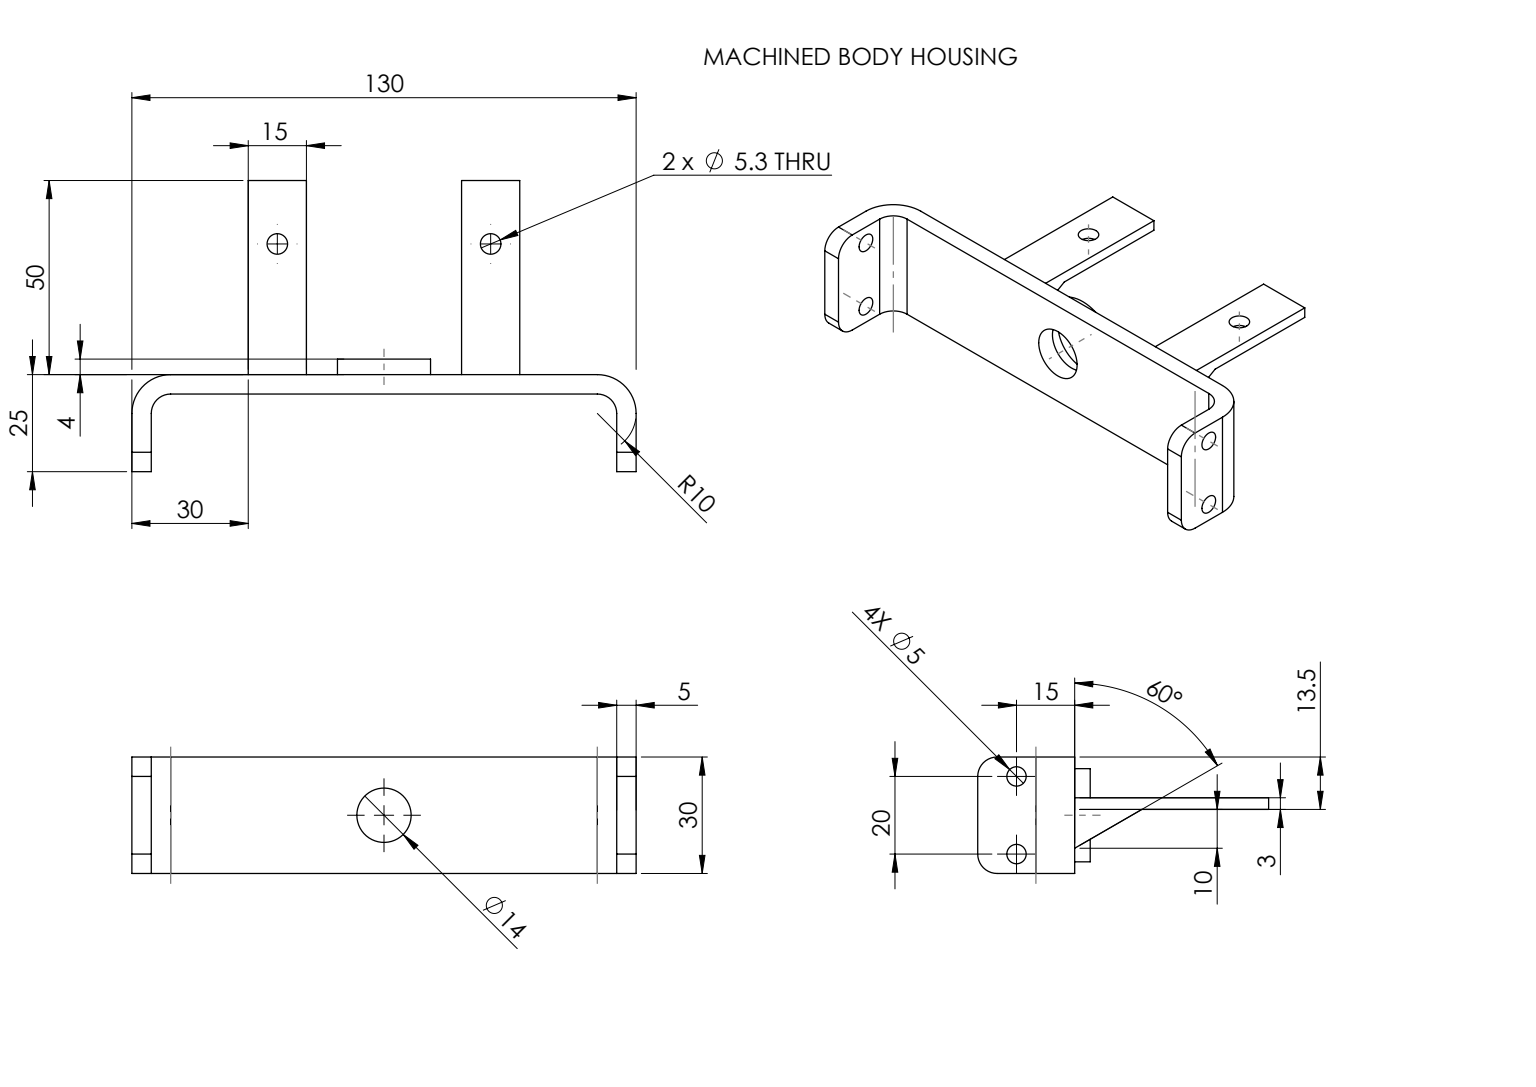
ISO-10303-21;
HEADER;
FILE_DESCRIPTION (('STEP AP214'),
    '1' );
FILE_NAME ('Machined Body Housing.step',
    '2026-10-08T13:46:47',
    ( '' ),
    ( '' ),
    'SwSTEP 2.0',
    'SolidWorks 2026',
    '' );
FILE_SCHEMA (( 'AUTOMOTIVE_DESIGN' ));
ENDSEC;

DATA;
#18=ORIENTED_EDGE ( 'NONE', *, *, #6198, .T. ) ;
#35=DIRECTION ( 'NONE',  ( -1.000000000000000000, 0.000000000000000000, 0.000000000000000000 ) ) ;
#69=PLANE ( 'NONE',  #9969 ) ;
#74=DIRECTION ( 'NONE',  ( 0.000000000000000000, 0.000000000000000000, -1.000000000000000000 ) ) ;
#91=EDGE_CURVE ( 'NONE', #13267, #15347, #17804, .T. ) ;
#103=DIRECTION ( 'NONE',  ( 1.224646799147353207E-16, -0.000000000000000000, 1.000000000000000000 ) ) ;
#106=EDGE_LOOP ( 'NONE', ( #16635, #20382, #2451, #21476 ) ) ;
#112=EDGE_CURVE ( 'NONE', #23518, #15611, #3206, .T. ) ;
#184=ORIENTED_EDGE ( 'NONE', *, *, #1140, .T. ) ;
#197=AXIS2_PLACEMENT_3D ( 'NONE', #16444, #18702, #9272 ) ;
#220=DIRECTION ( 'NONE',  ( 1.000000000000000000, -0.000000000000000000, -0.000000000000000000 ) ) ;
#235=CARTESIAN_POINT ( 'NONE',  ( -4.898587196589412829E-16, 0.000000000000000000, -4.000000000000000000 ) ) ;
#281=ORIENTED_EDGE ( 'NONE', *, *, #12290, .F. ) ;
#288=AXIS2_PLACEMENT_3D ( 'NONE', #14869, #22247, #466 ) ;
#296=DIRECTION ( 'NONE',  ( -0.000000000000000000, -1.000000000000000000, -0.000000000000000000 ) ) ;
#304=ORIENTED_EDGE ( 'NONE', *, *, #3176, .T. ) ;
#329=CARTESIAN_POINT ( 'NONE',  ( 27.50000000000000000, 1.500000000000003109, -33.66025403784446723 ) ) ;
#356=ORIENTED_EDGE ( 'NONE', *, *, #112, .T. ) ;
#362=DIRECTION ( 'NONE',  ( -0.000000000000000000, -1.000000000000000000, -0.000000000000000000 ) ) ;
#374=SHAPE_DEFINITION_REPRESENTATION ( #9332, #13579 ) ;
#392=CARTESIAN_POINT ( 'NONE',  ( -9.000000000000000000, 1.102182119232617714E-15, 1.102182119232617714E-15 ) ) ;
#407=DIRECTION ( 'NONE',  ( 0.000000000000000000, 0.000000000000000000, -1.000000000000000000 ) ) ;
#416=ADVANCED_FACE ( 'NONE', ( #532 ), #16955, .F. ) ;
#430=DIRECTION ( 'NONE',  ( 0.000000000000000000, 0.000000000000000000, -1.000000000000000000 ) ) ;
#463=CARTESIAN_POINT ( 'NONE',  ( 54.99999999999992895, 15.00000000000000000, 1.836970198721037478E-15 ) ) ;
#465=CARTESIAN_POINT ( 'NONE',  ( 9.000000000000000000, 0.000000000000000000, -4.000000000000000888 ) ) ;
#466=DIRECTION ( 'NONE',  ( -1.000000000000000000, 0.000000000000000000, 1.224646799147353207E-16 ) ) ;
#532=FACE_OUTER_BOUND ( 'NONE', #9949, .T. ) ;
#533=DIRECTION ( 'NONE',  ( 0.000000000000000000, 0.000000000000000000, 1.000000000000000000 ) ) ;
#547=EDGE_CURVE ( 'NONE', #15019, #16065, #20991, .T. ) ;
#548=FACE_OUTER_BOUND ( 'NONE', #8173, .T. ) ;
#559=DIRECTION ( 'NONE',  ( 0.000000000000000000, 0.000000000000000000, 1.000000000000000000 ) ) ;
#565=EDGE_LOOP ( 'NONE', ( #20115, #18574, #6373, #5474, #16669 ) ) ;
#589=VERTEX_POINT ( 'NONE', #18015 ) ;
#600=LINE ( 'NONE', #1067, #16099 ) ;
#621=DIRECTION ( 'NONE',  ( -0.000000000000000000, -1.000000000000000000, -0.000000000000000000 ) ) ;
#655=ORIENTED_EDGE ( 'NONE', *, *, #23127, .T. ) ;
#660=VERTEX_POINT ( 'NONE', #8631 ) ;
#677=DIRECTION ( 'NONE',  ( 0.000000000000000000, 0.000000000000000000, -1.000000000000000000 ) ) ;
#690=LINE ( 'NONE', #6575, #22493 ) ;
#693=ORIENTED_EDGE ( 'NONE', *, *, #18920, .T. ) ;
#697=CYLINDRICAL_SURFACE ( 'NONE', #7614, 2.500000000000002220 ) ;
#726=ORIENTED_EDGE ( 'NONE', *, *, #16884, .F. ) ;
#731=EDGE_LOOP ( 'NONE', ( #13217, #18222 ) ) ;
#733=EDGE_LOOP ( 'NONE', ( #2981, #9011 ) ) ;
#744=CYLINDRICAL_SURFACE ( 'NONE', #19501, 4.999999999999996447 ) ;
#754=VECTOR ( 'NONE', #8335, 1000.000000000000000 ) ;
#766=LINE ( 'NONE', #2680, #12959 ) ;
#770=VECTOR ( 'NONE', #3245, 1000.000000000000000 ) ;
#771=DIRECTION ( 'NONE',  ( 1.000000000000000000, 0.000000000000000000, 1.040834085586083271E-15 ) ) ;
#792=ORIENTED_EDGE ( 'NONE', *, *, #18099, .T. ) ;
#809=CARTESIAN_POINT ( 'NONE',  ( -65.00000000000000000, 9.999999999999998224, 14.99999999999999645 ) ) ;
#811=ORIENTED_EDGE ( 'NONE', *, *, #17044, .F. ) ;
#814=PLANE ( 'NONE',  #15172 ) ;
#831=DIRECTION ( 'NONE',  ( -1.000000000000000000, 0.000000000000000000, 1.239088197126290817E-16 ) ) ;
#897=ORIENTED_EDGE ( 'NONE', *, *, #13576, .T. ) ;
#900=DIRECTION ( 'NONE',  ( 1.000000000000000000, -0.000000000000000000, -1.224646799147353454E-16 ) ) ;
#912=CYLINDRICAL_SURFACE ( 'NONE', #1944, 5.000000000000000888 ) ;
#937=DIRECTION ( 'NONE',  ( 1.000000000000000000, 0.000000000000000000, 0.000000000000000000 ) ) ;
#941=VECTOR ( 'NONE', #12912, 1000.000000000000000 ) ;
#942=CARTESIAN_POINT ( 'NONE',  ( 54.99999999999994316, -8.499999999999944933, 1.836970198721036294E-15 ) ) ;
#954=EDGE_LOOP ( 'NONE', ( #23586, #9037, #13919, #18797 ) ) ;
#956=ORIENTED_EDGE ( 'NONE', *, *, #4066, .T. ) ;
#979=ORIENTED_EDGE ( 'NONE', *, *, #3064, .F. ) ;
#1004=EDGE_CURVE ( 'NONE', #5469, #15347, #8225, .T. ) ;
#1037=EDGE_CURVE ( 'NONE', #23404, #17536, #10992, .T. ) ;
#1043=ORIENTED_EDGE ( 'NONE', *, *, #13376, .T. ) ;
#1058=CARTESIAN_POINT ( 'NONE',  ( 65.00000000000000000, 9.999999999999998224, 19.99999999999999645 ) ) ;
#1061=LINE ( 'NONE', #942, #17401 ) ;
#1067=CARTESIAN_POINT ( 'NONE',  ( 54.99999999999992895, 15.00000000000000000, 1.836970198721037478E-15 ) ) ;
#1075=ORIENTED_EDGE ( 'NONE', *, *, #7209, .F. ) ;
#1081=LINE ( 'NONE', #13691, #1932 ) ;
#1094=ORIENTED_EDGE ( 'NONE', *, *, #6571, .T. ) ;
#1099=VECTOR ( 'NONE', #15927, 1000.000000000000000 ) ;
#1104=ORIENTED_EDGE ( 'NONE', *, *, #9994, .F. ) ;
#1133=CARTESIAN_POINT ( 'NONE',  ( -20.00000000000001066, 4.500000000000003553, -50.00000000000000000 ) ) ;
#1140=EDGE_CURVE ( 'NONE', #11837, #5919, #23282, .T. ) ;
#1143=AXIS2_PLACEMENT_3D ( 'NONE', #12271, #5410, #7224 ) ;
#1156=DIRECTION ( 'NONE',  ( 1.000000000000000000, -0.000000000000000000, -0.000000000000000000 ) ) ;
#1159=CARTESIAN_POINT ( 'NONE',  ( 60.00000000000000711, -15.00000000000000000, 19.99999999999999645 ) ) ;
#1201=EDGE_CURVE ( 'NONE', #19518, #3871, #23160, .T. ) ;
#1210=LINE ( 'NONE', #8194, #8825 ) ;
#1237=ORIENTED_EDGE ( 'NONE', *, *, #15576, .F. ) ;
#1268=LINE ( 'NONE', #10304, #1617 ) ;
#1284=CARTESIAN_POINT ( 'NONE',  ( 65.00000000000000000, -9.999999999999998224, 19.99999999999999645 ) ) ;
#1297=VERTEX_POINT ( 'NONE', #7729 ) ;
#1305=ORIENTED_EDGE ( 'NONE', *, *, #8806, .T. ) ;
#1313=DIRECTION ( 'NONE',  ( 1.000000000000000000, 0.000000000000000000, 0.000000000000000000 ) ) ;
#1320=DIRECTION ( 'NONE',  ( 1.224646799147353207E-16, -0.000000000000000000, 1.000000000000000000 ) ) ;
#1357=VERTEX_POINT ( 'NONE', #22052 ) ;
#1379=LINE ( 'NONE', #7284, #5572 ) ;
#1382=PLANE ( 'NONE',  #19705 ) ;
#1426=AXIS2_PLACEMENT_3D ( 'NONE', #20889, #22335, #13514 ) ;
#1431=DIRECTION ( 'NONE',  ( 1.224646799147353207E-16, -0.000000000000000000, 1.000000000000000000 ) ) ;
#1462=EDGE_CURVE ( 'NONE', #20146, #12336, #3240, .T. ) ;
#1464=CARTESIAN_POINT ( 'NONE',  ( 20.00000000000000000, 1.500000000000003109, -17.32050807568893092 ) ) ;
#1471=EDGE_CURVE ( 'NONE', #16384, #8981, #8772, .T. ) ;
#1475=AXIS2_PLACEMENT_3D ( 'NONE', #8775, #10591, #19885 ) ;
#1498=CIRCLE ( 'NONE', #10721, 2.499999999999998668 ) ;
#1514=DIRECTION ( 'NONE',  ( 1.000000000000000000, 4.625929269271486900E-16, 0.000000000000000000 ) ) ;
#1520=ORIENTED_EDGE ( 'NONE', *, *, #23567, .F. ) ;
#1528=DIRECTION ( 'NONE',  ( -1.224646799147353207E-16, 0.000000000000000000, -1.000000000000000000 ) ) ;
#1542=( NAMED_UNIT ( * ) PLANE_ANGLE_UNIT ( ) SI_UNIT ( $, .RADIAN. ) );
#1561=DIRECTION ( 'NONE',  ( -1.000000000000000000, 0.000000000000000000, 0.000000000000000000 ) ) ;
#1569=ADVANCED_FACE ( 'NONE', ( #21794 ), #6968, .T. ) ;
#1582=ADVANCED_FACE ( 'NONE', ( #23477 ), #14407, .F. ) ;
#1585=CARTESIAN_POINT ( 'NONE',  ( -20.00000000000001066, 4.500000000000003553, -50.00000000000000000 ) ) ;
#1617=VECTOR ( 'NONE', #1156, 1000.000000000000000 ) ;
#1626=CARTESIAN_POINT ( 'NONE',  ( -65.00000000000000000, 9.999999999999998224, 25.00000000000001421 ) ) ;
#1630=CARTESIAN_POINT ( 'NONE',  ( 65.00000000000000000, 15.00000000000000000, 10.00000000000007105 ) ) ;
#1633=LINE ( 'NONE', #12448, #22458 ) ;
#1662=FACE_OUTER_BOUND ( 'NONE', #23691, .T. ) ;
#1670=VECTOR ( 'NONE', #16250, 1000.000000000000000 ) ;
#1675=ADVANCED_FACE ( 'NONE', ( #12532 ), #16223, .F. ) ;
#1682=DIRECTION ( 'NONE',  ( -1.000000000000000000, 0.000000000000000000, 1.224646799147353207E-16 ) ) ;
#1694=CYLINDRICAL_SURFACE ( 'NONE', #12537, 2.649999999999999467 ) ;
#1722=CARTESIAN_POINT ( 'NONE',  ( -54.99999999999992895, 15.00000000000000000, 5.000000000000015987 ) ) ;
#1725=PLANE ( 'NONE',  #11097 ) ;
#1726=CARTESIAN_POINT ( 'NONE',  ( 55.00000000000000711, 15.00000000000000000, 10.00000000000000000 ) ) ;
#1730=EDGE_CURVE ( 'NONE', #18272, #11666, #15988, .T. ) ;
#1739=EDGE_CURVE ( 'NONE', #7101, #5362, #20376, .T. ) ;
#1747=DIRECTION ( 'NONE',  ( 0.000000000000000000, 0.000000000000000000, 1.000000000000000000 ) ) ;
#1748=CARTESIAN_POINT ( 'NONE',  ( 65.00000000000000000, -10.00000000000000178, 12.49999999999999467 ) ) ;
#1750=ORIENTED_EDGE ( 'NONE', *, *, #9693, .F. ) ;
#1767=DIRECTION ( 'NONE',  ( 1.224646799147353207E-16, -0.000000000000000000, 1.000000000000000000 ) ) ;
#1789=CARTESIAN_POINT ( 'NONE',  ( -4.898587196589412829E-16, 0.000000000000000000, -4.000000000000000000 ) ) ;
#1796=CARTESIAN_POINT ( 'NONE',  ( -35.00000000000000000, 4.500000000000003553, 4.286263797015736496E-15 ) ) ;
#1813=DIRECTION ( 'NONE',  ( 0.000000000000000000, 0.000000000000000000, -1.000000000000000000 ) ) ;
#1840=ORIENTED_EDGE ( 'NONE', *, *, #8806, .F. ) ;
#1841=FACE_OUTER_BOUND ( 'NONE', #21249, .T. ) ;
#1844=EDGE_CURVE ( 'NONE', #13106, #19458, #9139, .T. ) ;
#1850=CARTESIAN_POINT ( 'NONE',  ( -54.99999999999992895, 15.00000000000000000, 5.000000000000015987 ) ) ;
#1866=VECTOR ( 'NONE', #21905, 1000.000000000000000 ) ;
#1873=EDGE_CURVE ( 'NONE', #19365, #1924, #15036, .T. ) ;
#1879=DIRECTION ( 'NONE',  ( -1.000000000000000000, 0.000000000000000000, 9.637352644315595243E-17 ) ) ;
#1889=AXIS2_PLACEMENT_3D ( 'NONE', #22318, #533, #7508 ) ;
#1913=VERTEX_POINT ( 'NONE', #16458 ) ;
#1919=DIRECTION ( 'NONE',  ( -1.000000000000000000, 0.000000000000000000, 1.445602896647339163E-16 ) ) ;
#1924=VERTEX_POINT ( 'NONE', #392 ) ;
#1929=PRODUCT_CONTEXT ( 'NONE', #12856, 'mechanical' ) ;
#1930=DIRECTION ( 'NONE',  ( -1.224646799147353207E-16, 0.000000000000000000, -1.000000000000000000 ) ) ;
#1932=VECTOR ( 'NONE', #20953, 1000.000000000000000 ) ;
#1933=ORIENTED_EDGE ( 'NONE', *, *, #10842, .F. ) ;
#1944=AXIS2_PLACEMENT_3D ( 'NONE', #8248, #20792, #13523 ) ;
#1961=CARTESIAN_POINT ( 'NONE',  ( -4.898587196589412829E-16, 0.000000000000000000, -4.000000000000000000 ) ) ;
#1962=CARTESIAN_POINT ( 'NONE',  ( 20.00000000000000355, 4.500000000000003553, -2.449293598294706907E-15 ) ) ;
#1967=CARTESIAN_POINT ( 'NONE',  ( -27.50000000000000711, 1.500000000000003109, -31.01025403784446510 ) ) ;
#1979=EDGE_LOOP ( 'NONE', ( #21980, #9928, #1104, #8440 ) ) ;
#1997=DIRECTION ( 'NONE',  ( 0.000000000000000000, 0.000000000000000000, 1.000000000000000000 ) ) ;
#2012=LINE ( 'NONE', #16764, #18322 ) ;
#2017=DIRECTION ( 'NONE',  ( 0.000000000000000000, 0.000000000000000000, -1.000000000000000000 ) ) ;
#2020=VERTEX_POINT ( 'NONE', #8302 ) ;
#2023=CARTESIAN_POINT ( 'NONE',  ( -60.00000000000000711, -15.00000000000000000, 10.00000000000004974 ) ) ;
#2069=DIRECTION ( 'NONE',  ( 0.000000000000000000, 0.000000000000000000, 1.000000000000000000 ) ) ;
#2100=ORIENTED_EDGE ( 'NONE', *, *, #3101, .T. ) ;
#2111=AXIS2_PLACEMENT_3D ( 'NONE', #14632, #9595, #21892 ) ;
#2141=ADVANCED_FACE ( 'NONE', ( #6972 ), #5163, .F. ) ;
#2155=EDGE_LOOP ( 'NONE', ( #7268, #12154, #13017, #8583 ) ) ;
#2203=AXIS2_PLACEMENT_3D ( 'NONE', #4413, #11869, #6458 ) ;
#2223=DIRECTION ( 'NONE',  ( -0.000000000000000000, -1.000000000000000000, -0.000000000000000000 ) ) ;
#2236=VERTEX_POINT ( 'NONE', #7003 ) ;
#2271=DIRECTION ( 'NONE',  ( 0.000000000000000000, 0.000000000000000000, -1.000000000000000000 ) ) ;
#2290=EDGE_LOOP ( 'NONE', ( #6796, #9438 ) ) ;
#2329=LINE ( 'NONE', #7976, #16409 ) ;
#2351=LINE ( 'NONE', #15558, #6078 ) ;
#2372=VERTEX_POINT ( 'NONE', #4318 ) ;
#2389=DIRECTION ( 'NONE',  ( 1.000000000000000000, 0.000000000000000000, 0.000000000000000000 ) ) ;
#2406=EDGE_LOOP ( 'NONE', ( #2495, #956 ) ) ;
#2426=ORIENTED_EDGE ( 'NONE', *, *, #14982, .T. ) ;
#2451=ORIENTED_EDGE ( 'NONE', *, *, #3652, .F. ) ;
#2467=VECTOR ( 'NONE', #12355, 1000.000000000000000 ) ;
#2495=ORIENTED_EDGE ( 'NONE', *, *, #15806, .T. ) ;
#2511=DIRECTION ( 'NONE',  ( 0.000000000000000000, 0.000000000000000000, 1.000000000000000000 ) ) ;
#2536=DIRECTION ( 'NONE',  ( 1.224646799147353207E-16, -0.000000000000000000, 1.000000000000000000 ) ) ;
#2539=ORIENTED_EDGE ( 'NONE', *, *, #16677, .T. ) ;
#2560=PLANE ( 'NONE',  #21397 ) ;
#2586=CARTESIAN_POINT ( 'NONE',  ( -20.00000000000000711, 1.500000000000003109, -17.32050807568893092 ) ) ;
#2609=CIRCLE ( 'NONE', #5678, 2.500000000000000444 ) ;
#2633=DIRECTION ( 'NONE',  ( 0.000000000000000000, -1.000000000000000000, 0.000000000000000000 ) ) ;
#2634=PRODUCT ( 'Machined Body Housing', 'Machined Body Housing', '', ( #1929 ) ) ;
#2650=AXIS2_PLACEMENT_3D ( 'NONE', #8276, #2970, #4899 ) ;
#2673=ORIENTED_EDGE ( 'NONE', *, *, #17745, .F. ) ;
#2680=CARTESIAN_POINT ( 'NONE',  ( 34.99999999999999289, 16.40063509461080571, -43.12916512459904794 ) ) ;
#2701=VERTEX_POINT ( 'NONE', #12627 ) ;
#2704=LINE ( 'NONE', #18874, #16750 ) ;
#2721=CARTESIAN_POINT ( 'NONE',  ( 60.00000000000000000, 9.999999999999998224, 14.99999999999999645 ) ) ;
#2722=DIRECTION ( 'NONE',  ( 0.000000000000000000, 0.000000000000000000, -1.000000000000000000 ) ) ;
#2725=DIRECTION ( 'NONE',  ( -1.224646799147353207E-16, 0.000000000000000000, -1.000000000000000000 ) ) ;
#2736=EDGE_CURVE ( 'NONE', #15611, #13122, #20088, .T. ) ;
#2753=CARTESIAN_POINT ( 'NONE',  ( 20.00000000000000355, 4.500000000000003553, -2.449293598294706907E-15 ) ) ;
#2765=CIRCLE ( 'NONE', #11983, 2.500000000000000444 ) ;
#2802=CARTESIAN_POINT ( 'NONE',  ( -65.00000000000000000, 15.00000000000000000, 10.00000000000008882 ) ) ;
#2832=LINE ( 'NONE', #6210, #21016 ) ;
#2845=CIRCLE ( 'NONE', #14351, 7.000000000000000000 ) ;
#2852=CYLINDRICAL_SURFACE ( 'NONE', #16801, 5.000000000000000888 ) ;
#2863=CARTESIAN_POINT ( 'NONE',  ( -20.00000000000000355, 4.500000000000003553, 2.449293598294706907E-15 ) ) ;
#2872=ORIENTED_EDGE ( 'NONE', *, *, #10537, .F. ) ;
#2883=CIRCLE ( 'NONE', #5960, 2.500000000000000444 ) ;
#2884=VECTOR ( 'NONE', #10996, 1000.000000000000000 ) ;
#2902=EDGE_LOOP ( 'NONE', ( #16031, #23184 ) ) ;
#2912=CARTESIAN_POINT ( 'NONE',  ( -20.00000000000001066, 4.500000000000003553, -50.00000000000000000 ) ) ;
#2939=DIRECTION ( 'NONE',  ( -1.000000000000000000, 0.000000000000000000, 0.000000000000000000 ) ) ;
#2967=VERTEX_POINT ( 'NONE', #10539 ) ;
#2970=DIRECTION ( 'NONE',  ( -1.224646799147353207E-16, 0.000000000000000000, -1.000000000000000000 ) ) ;
#2971=DIRECTION ( 'NONE',  ( 4.625929269271486900E-16, -1.000000000000000000, -5.665129472695380173E-32 ) ) ;
#2974=DIRECTION ( 'NONE',  ( 1.224646799147353207E-16, -0.000000000000000000, 1.000000000000000000 ) ) ;
#2976=ORIENTED_EDGE ( 'NONE', *, *, #19049, .T. ) ;
#2981=ORIENTED_EDGE ( 'NONE', *, *, #3861, .T. ) ;
#2990=VERTEX_POINT ( 'NONE', #17473 ) ;
#2999=CIRCLE ( 'NONE', #8002, 5.000000000000004441 ) ;
#3032=DIRECTION ( 'NONE',  ( -1.000000000000000000, -4.625929269271486900E-16, 1.224646799147353207E-16 ) ) ;
#3034=EDGE_CURVE ( 'NONE', #11666, #22477, #2765, .T. ) ;
#3043=EDGE_CURVE ( 'NONE', #9561, #17175, #8918, .T. ) ;
#3044=CARTESIAN_POINT ( 'NONE',  ( -6.123233995736766085E-15, 0.000000000000000000, -50.00000000000000000 ) ) ;
#3048=DIRECTION ( 'NONE',  ( 1.224646799147353207E-16, -0.000000000000000000, 1.000000000000000000 ) ) ;
#3060=CIRCLE ( 'NONE', #9211, 2.500000000000000444 ) ;
#3062=UNCERTAINTY_MEASURE_WITH_UNIT (LENGTH_MEASURE( 1.000000000000000082E-05 ), #21533, 'distance_accuracy_value', 'NONE');
#3064=EDGE_CURVE ( 'NONE', #21915, #22477, #1268, .T. ) ;
#3085=CARTESIAN_POINT ( 'NONE',  ( 60.00000000000000711, 15.00000000000000000, 10.00000000000007105 ) ) ;
#3088=ORIENTED_EDGE ( 'NONE', *, *, #20465, .T. ) ;
#3101=EDGE_CURVE ( 'NONE', #17422, #16065, #23187, .T. ) ;
#3107=ORIENTED_EDGE ( 'NONE', *, *, #19599, .F. ) ;
#3111=CARTESIAN_POINT ( 'NONE',  ( 0.000000000000000000, 0.000000000000000000, 0.000000000000000000 ) ) ;
#3119=CARTESIAN_POINT ( 'NONE',  ( -4.898587196589412829E-16, 0.000000000000000000, -4.000000000000000000 ) ) ;
#3161=ORIENTED_EDGE ( 'NONE', *, *, #22071, .T. ) ;
#3176=EDGE_CURVE ( 'NONE', #9843, #3750, #11234, .T. ) ;
#3188=CARTESIAN_POINT ( 'NONE',  ( 54.99999999999996447, 15.00000000000000000, 5.000000000000003553 ) ) ;
#3206=CIRCLE ( 'NONE', #20788, 10.00000000000000178 ) ;
#3240=LINE ( 'NONE', #5156, #6403 ) ;
#3245=DIRECTION ( 'NONE',  ( 1.000000000000000000, -0.000000000000000000, -0.000000000000000000 ) ) ;
#3252=EDGE_LOOP ( 'NONE', ( #9859, #14478 ) ) ;
#3260=DIRECTION ( 'NONE',  ( 4.625929269271486900E-16, -1.000000000000000000, -5.665129472695380173E-32 ) ) ;
#3261=VECTOR ( 'NONE', #12153, 1000.000000000000000 ) ;
#3263=AXIS2_PLACEMENT_3D ( 'NONE', #15448, #22715, #20682 ) ;
#3271=AXIS2_PLACEMENT_3D ( 'NONE', #809, #13421, #2722 ) ;
#3284=DIRECTION ( 'NONE',  ( 1.000000000000000000, 4.625929269271485914E-16, -1.224646799147353454E-16 ) ) ;
#3293=DIRECTION ( 'NONE',  ( -1.224646799147353207E-16, 0.000000000000000000, -1.000000000000000000 ) ) ;
#3323=VECTOR ( 'NONE', #3284, 1000.000000000000000 ) ;
#3338=VECTOR ( 'NONE', #14817, 1000.000000000000000 ) ;
#3353=CARTESIAN_POINT ( 'NONE',  ( 0.000000000000000000, 0.000000000000000000, 1.734723475976807094E-15 ) ) ;
#3381=CARTESIAN_POINT ( 'NONE',  ( 19.99999999999999645, 4.500000000000003553, -50.00000000000000000 ) ) ;
#3382=ORIENTED_EDGE ( 'NONE', *, *, #11929, .T. ) ;
#3383=CARTESIAN_POINT ( 'NONE',  ( -65.00000000000000000, 9.999999999999998224, 12.49999999999999289 ) ) ;
#3399=EDGE_CURVE ( 'NONE', #17589, #22866, #10576, .T. ) ;
#3418=FACE_OUTER_BOUND ( 'NONE', #19840, .T. ) ;
#3434=DIRECTION ( 'NONE',  ( 1.000000000000000000, 0.000000000000000000, -1.224646799147353207E-16 ) ) ;
#3452=CARTESIAN_POINT ( 'NONE',  ( 65.00000000000000000, 9.999999999999998224, 14.99999999999999645 ) ) ;
#3464=ORIENTED_EDGE ( 'NONE', *, *, #6828, .F. ) ;
#3489=DIRECTION ( 'NONE',  ( -1.000000000000000000, 0.000000000000000000, 0.000000000000000000 ) ) ;
#3495=APPLICATION_CONTEXT ( 'automotive_design' ) ;
#3507=DIRECTION ( 'NONE',  ( -0.000000000000000000, -0.000000000000000000, 1.000000000000000000 ) ) ;
#3524=EDGE_LOOP ( 'NONE', ( #18220, #11976 ) ) ;
#3530=ORIENTED_EDGE ( 'NONE', *, *, #6636, .T. ) ;
#3557=EDGE_LOOP ( 'NONE', ( #3991, #655 ) ) ;
#3561=ADVANCED_FACE ( 'NONE', ( #7547, #10918 ), #11268, .T. ) ;
#3570=DIRECTION ( 'NONE',  ( 1.000000000000000000, -0.000000000000000000, -0.000000000000000000 ) ) ;
#3609=DIRECTION ( 'NONE',  ( 1.000000000000000000, 0.000000000000000000, -1.224646799147353207E-16 ) ) ;
#3612=DIRECTION ( 'NONE',  ( -0.000000000000000000, -0.000000000000000000, 1.000000000000000000 ) ) ;
#3616=AXIS2_PLACEMENT_3D ( 'NONE', #20348, #19888, #3489 ) ;
#3650=LINE ( 'NONE', #1850, #21769 ) ;
#3652=EDGE_CURVE ( 'NONE', #7101, #9090, #22392, .T. ) ;
#3656=AXIS2_PLACEMENT_3D ( 'NONE', #21284, #10210, #2511 ) ;
#3657=DIRECTION ( 'NONE',  ( 0.000000000000000000, 0.000000000000000000, 1.000000000000000000 ) ) ;
#3659=DIRECTION ( 'NONE',  ( 0.000000000000000000, -0.000000000000000000, 1.000000000000000000 ) ) ;
#3663=ORIENTED_EDGE ( 'NONE', *, *, #1140, .F. ) ;
#3666=CARTESIAN_POINT ( 'NONE',  ( 20.00000000000000000, 1.500000000000003109, -17.32050807568893092 ) ) ;
#3682=CARTESIAN_POINT ( 'NONE',  ( -20.00000000000000711, 1.500000000000003109, -17.32050807568893092 ) ) ;
#3688=EDGE_CURVE ( 'NONE', #11955, #2020, #16528, .T. ) ;
#3728=CARTESIAN_POINT ( 'NONE',  ( 7.000000000000000000, 0.000000000000000000, 1.734723475976807094E-15 ) ) ;
#3743=VERTEX_POINT ( 'NONE', #4650 ) ;
#3750=VERTEX_POINT ( 'NONE', #20914 ) ;
#3769=LINE ( 'NONE', #15301, #16820 ) ;
#3776=CARTESIAN_POINT ( 'NONE',  ( 19.99999999999999645, 1.500000000000003109, -50.00000000000000000 ) ) ;
#3800=ADVANCED_FACE ( 'NONE', ( #22968 ), #814, .T. ) ;
#3808=AXIS2_PLACEMENT_3D ( 'NONE', #3452, #17945, #14727 ) ;
#3831=DIRECTION ( 'NONE',  ( -0.000000000000000000, -1.000000000000000000, -0.000000000000000000 ) ) ;
#3836=VECTOR ( 'NONE', #1682, 1000.000000000000000 ) ;
#3861=EDGE_CURVE ( 'NONE', #22477, #11666, #2883, .T. ) ;
#3871=VERTEX_POINT ( 'NONE', #15580 ) ;
#3894=EDGE_CURVE ( 'NONE', #7429, #13541, #9042, .T. ) ;
#3896=ORIENTED_EDGE ( 'NONE', *, *, #4429, .T. ) ;
#3912=VERTEX_POINT ( 'NONE', #23322 ) ;
#3922=EDGE_LOOP ( 'NONE', ( #18403, #14686, #11774, #18278 ) ) ;
#3927=AXIS2_PLACEMENT_3D ( 'NONE', #13450, #22511, #22024 ) ;
#3944=CARTESIAN_POINT ( 'NONE',  ( 60.00000000000000000, -10.00000000000000178, 14.99999999999999467 ) ) ;
#3962=ORIENTED_EDGE ( 'NONE', *, *, #23567, .T. ) ;
#3991=ORIENTED_EDGE ( 'NONE', *, *, #9236, .T. ) ;
#4001=CIRCLE ( 'NONE', #5146, 2.649999999999999467 ) ;
#4012=VECTOR ( 'NONE', #21254, 1000.000000000000000 ) ;
#4016=CARTESIAN_POINT ( 'NONE',  ( 54.99999999999996447, 15.00000000000000000, 5.000000000000003553 ) ) ;
#4049=CARTESIAN_POINT ( 'NONE',  ( 65.00000000000000000, -15.00000000000000000, 19.99999999999999645 ) ) ;
#4066=EDGE_CURVE ( 'NONE', #2967, #17589, #20221, .T. ) ;
#4103=EDGE_CURVE ( 'NONE', #16245, #5234, #5917, .T. ) ;
#4112=ORIENTED_EDGE ( 'NONE', *, *, #13576, .F. ) ;
#4159=CARTESIAN_POINT ( 'NONE',  ( -27.50000000000000711, 1.500000000000003109, -31.01025403784446510 ) ) ;
#4166=DIRECTION ( 'NONE',  ( 0.000000000000000000, 0.000000000000000000, -1.000000000000000000 ) ) ;
#4246=DIRECTION ( 'NONE',  ( -1.224646799147353207E-16, 0.000000000000000000, -1.000000000000000000 ) ) ;
#4270=CARTESIAN_POINT ( 'NONE',  ( 34.99999999999999289, 4.500000000000009770, -50.00000000000000711 ) ) ;
#4275=UNCERTAINTY_MEASURE_WITH_UNIT (LENGTH_MEASURE( 1.000000000000000082E-05 ), #10865, 'distance_accuracy_value', 'NONE');
#4281=FACE_BOUND ( 'NONE', #2290, .T. ) ;
#4291=FACE_OUTER_BOUND ( 'NONE', #2155, .T. ) ;
#4296=CARTESIAN_POINT ( 'NONE',  ( -60.00000000000000711, -10.00000000000000178, 14.99999999999999467 ) ) ;
#4310=CARTESIAN_POINT ( 'NONE',  ( -35.00000000000000711, 4.500000000000003553, -49.99999999999999289 ) ) ;
#4318=CARTESIAN_POINT ( 'NONE',  ( -35.00000000000000711, 1.500000000000003109, -49.99999999999999289 ) ) ;
#4393=AXIS2_PLACEMENT_3D ( 'NONE', #3682, #7538, #13062 ) ;
#4408=FACE_OUTER_BOUND ( 'NONE', #18514, .T. ) ;
#4413=CARTESIAN_POINT ( 'NONE',  ( 0.000000000000000000, 0.000000000000000000, 0.000000000000000000 ) ) ;
#4429=EDGE_CURVE ( 'NONE', #2372, #15450, #8304, .T. ) ;
#4492=CARTESIAN_POINT ( 'NONE',  ( 60.00000000000000000, 9.999999999999998224, 12.49999999999999289 ) ) ;
#4502=VERTEX_POINT ( 'NONE', #23124 ) ;
#4504=( GEOMETRIC_REPRESENTATION_CONTEXT ( 3 ) GLOBAL_UNCERTAINTY_ASSIGNED_CONTEXT ( ( #4275 ) ) GLOBAL_UNIT_ASSIGNED_CONTEXT ( ( #10865, #7140, #7018 ) ) REPRESENTATION_CONTEXT ( 'NONE', 'WORKASPACE' ) );
#4541=EDGE_CURVE ( 'NONE', #7429, #5469, #8903, .T. ) ;
#4568=ORIENTED_EDGE ( 'NONE', *, *, #15106, .T. ) ;
#4576=AXIS2_PLACEMENT_3D ( 'NONE', #11141, #18415, #5247 ) ;
#4589=ORIENTED_EDGE ( 'NONE', *, *, #12262, .T. ) ;
#4603=EDGE_CURVE ( 'NONE', #6374, #3871, #12508, .T. ) ;
#4610=CARTESIAN_POINT ( 'NONE',  ( -20.00000000000001066, 1.500000000000003109, -50.00000000000000000 ) ) ;
#4618=FACE_OUTER_BOUND ( 'NONE', #20979, .T. ) ;
#4635=EDGE_CURVE ( 'NONE', #16065, #8909, #15960, .T. ) ;
#4650=CARTESIAN_POINT ( 'NONE',  ( -65.00000000000000000, -15.00000000000000000, 20.00000000000001421 ) ) ;
#4652=ORIENTED_EDGE ( 'NONE', *, *, #11929, .F. ) ;
#4667=DIRECTION ( 'NONE',  ( -1.224646799147353207E-16, 0.000000000000000000, -1.000000000000000000 ) ) ;
#4689=VECTOR ( 'NONE', #23241, 1000.000000000000000 ) ;
#4692=EDGE_CURVE ( 'NONE', #2020, #1924, #14285, .T. ) ;
#4710=CARTESIAN_POINT ( 'NONE',  ( -65.00000000000000000, 9.999999999999998224, 25.00000000000001421 ) ) ;
#4719=FACE_OUTER_BOUND ( 'NONE', #15486, .T. ) ;
#4784=CARTESIAN_POINT ( 'NONE',  ( 60.00000000000000711, 9.999999999999998224, 24.99999999999999645 ) ) ;
#4817=ORIENTED_EDGE ( 'NONE', *, *, #16677, .F. ) ;
#4822=VERTEX_POINT ( 'NONE', #4784 ) ;
#4825=EDGE_LOOP ( 'NONE', ( #10672, #20703, #8293, #4112 ) ) ;
#4832=EDGE_CURVE ( 'NONE', #3912, #7937, #21240, .T. ) ;
#4857=ORIENTED_EDGE ( 'NONE', *, *, #12635, .T. ) ;
#4863=VECTOR ( 'NONE', #12869, 1000.000000000000000 ) ;
#4866=CARTESIAN_POINT ( 'NONE',  ( -60.00000000000000711, -15.00000000000000000, 10.00000000000008882 ) ) ;
#4874=ORIENTED_EDGE ( 'NONE', *, *, #18393, .F. ) ;
#4877=CARTESIAN_POINT ( 'NONE',  ( 0.000000000000000000, 0.000000000000000000, 5.000000000000008882 ) ) ;
#4888=VECTOR ( 'NONE', #6882, 1000.000000000000000 ) ;
#4899=DIRECTION ( 'NONE',  ( -1.000000000000000000, 0.000000000000000000, 1.445602896647339163E-16 ) ) ;
#4906=ORIENTED_EDGE ( 'NONE', *, *, #12223, .T. ) ;
#4916=DIRECTION ( 'NONE',  ( -1.000000000000000000, 0.000000000000000000, 1.224646799147353207E-16 ) ) ;
#4939=VERTEX_POINT ( 'NONE', #10089 ) ;
#4957=DIRECTION ( 'NONE',  ( -0.000000000000000000, -1.000000000000000000, -0.000000000000000000 ) ) ;
#4971=CARTESIAN_POINT ( 'NONE',  ( 20.00000000000000355, 4.500000000000003553, -2.449293598294706907E-15 ) ) ;
#4973=ORIENTED_EDGE ( 'NONE', *, *, #3043, .F. ) ;
#4991=CIRCLE ( 'NONE', #1143, 2.499999999999998668 ) ;
#4994=PLANE ( 'NONE',  #10743 ) ;
#5007=ORIENTED_EDGE ( 'NONE', *, *, #23465, .F. ) ;
#5027=ORIENTED_EDGE ( 'NONE', *, *, #23127, .F. ) ;
#5049=CARTESIAN_POINT ( 'NONE',  ( 19.99999999999999645, 1.500000000000003109, -50.00000000000000000 ) ) ;
#5081=CARTESIAN_POINT ( 'NONE',  ( -27.50000000000000711, 4.500000000000003553, -33.66025403784446723 ) ) ;
#5102=DIRECTION ( 'NONE',  ( 0.000000000000000000, -1.000000000000000000, -0.000000000000000000 ) ) ;
#5117=ADVANCED_FACE ( 'NONE', ( #4291 ), #19133, .F. ) ;
#5127=EDGE_CURVE ( 'NONE', #23404, #17175, #13529, .T. ) ;
#5136=CARTESIAN_POINT ( 'NONE',  ( 19.99999999999999645, 4.500000000000003553, -50.00000000000000000 ) ) ;
#5146=AXIS2_PLACEMENT_3D ( 'NONE', #5081, #8694, #9054 ) ;
#5156=CARTESIAN_POINT ( 'NONE',  ( 12.00000000000000000, 0.000000000000000000, -4.000000000000001776 ) ) ;
#5163=PLANE ( 'NONE',  #20370 ) ;
#5176=ORIENTED_EDGE ( 'NONE', *, *, #16388, .F. ) ;
#5193=VECTOR ( 'NONE', #10534, 1000.000000000000000 ) ;
#5196=CARTESIAN_POINT ( 'NONE',  ( -20.00000000000001066, 1.500000000000003109, -50.00000000000000000 ) ) ;
#5208=ORIENTED_EDGE ( 'NONE', *, *, #6571, .F. ) ;
#5234=VERTEX_POINT ( 'NONE', #1748 ) ;
#5247=DIRECTION ( 'NONE',  ( 0.000000000000000000, 0.000000000000000000, -1.000000000000000000 ) ) ;
#5249=DIRECTION ( 'NONE',  ( 1.000000000000000000, 3.273063162220391312E-16, 0.000000000000000000 ) ) ;
#5251=VECTOR ( 'NONE', #11361, 1000.000000000000114 ) ;
#5254=ADVANCED_FACE ( 'NONE', ( #12444, #19594 ), #1382, .F. ) ;
#5260=( NAMED_UNIT ( * ) SI_UNIT ( $, .STERADIAN. ) SOLID_ANGLE_UNIT ( ) );
#5269=ORIENTED_EDGE ( 'NONE', *, *, #4103, .F. ) ;
#5275=AXIS2_PLACEMENT_3D ( 'NONE', #16971, #7872, #15193 ) ;
#5278=DIRECTION ( 'NONE',  ( 1.224646799147353207E-16, -0.000000000000000000, 1.000000000000000000 ) ) ;
#5300=ORIENTED_EDGE ( 'NONE', *, *, #22976, .F. ) ;
#5301=CARTESIAN_POINT ( 'NONE',  ( 27.50000000000000000, 4.500000000000006217, -33.66025403784446723 ) ) ;
#5303=VERTEX_POINT ( 'NONE', #8974 ) ;
#5306=CIRCLE ( 'NONE', #8384, 5.000000000000000888 ) ;
#5340=CARTESIAN_POINT ( 'NONE',  ( -60.00000000000000711, -15.00000000000000000, 20.00000000000001421 ) ) ;
#5351=LINE ( 'NONE', #9314, #15340 ) ;
#5362=VERTEX_POINT ( 'NONE', #10884 ) ;
#5387=CYLINDRICAL_SURFACE ( 'NONE', #12458, 2.499999999999998668 ) ;
#5404=EDGE_CURVE ( 'NONE', #7665, #13106, #12334, .T. ) ;
#5410=DIRECTION ( 'NONE',  ( 1.000000000000000000, -0.000000000000000000, -0.000000000000000000 ) ) ;
#5429=ADVANCED_FACE ( 'NONE', ( #20534 ), #13269, .F. ) ;
#5469=VERTEX_POINT ( 'NONE', #9315 ) ;
#5474=ORIENTED_EDGE ( 'NONE', *, *, #17611, .F. ) ;
#5495=VECTOR ( 'NONE', #18311, 1000.000000000000000 ) ;
#5530=CARTESIAN_POINT ( 'NONE',  ( -35.00000000000000711, 4.500000000000003553, -49.99999999999999289 ) ) ;
#5548=PLANE ( 'NONE',  #8428 ) ;
#5566=DIRECTION ( 'NONE',  ( 0.000000000000000000, 0.000000000000000000, -1.000000000000000000 ) ) ;
#5572=VECTOR ( 'NONE', #8850, 1000.000000000000000 ) ;
#5582=DIRECTION ( 'NONE',  ( 1.000000000000000000, 0.000000000000000000, -0.000000000000000000 ) ) ;
#5603=ORIENTED_EDGE ( 'NONE', *, *, #17224, .T. ) ;
#5617=CARTESIAN_POINT ( 'NONE',  ( -27.50000000000000711, 1.500000000000003109, -33.66025403784446723 ) ) ;
#5629=PLANE ( 'NONE',  #16727 ) ;
#5678=AXIS2_PLACEMENT_3D ( 'NONE', #21988, #21639, #9099 ) ;
#5699=EDGE_CURVE ( 'NONE', #6393, #16436, #23206, .T. ) ;
#5714=CIRCLE ( 'NONE', #4576, 2.500000000000002220 ) ;
#5723=ORIENTED_EDGE ( 'NONE', *, *, #16855, .T. ) ;
#5725=DIRECTION ( 'NONE',  ( 0.000000000000000000, -1.000000000000000000, -0.000000000000000000 ) ) ;
#5752=DIRECTION ( 'NONE',  ( 0.000000000000000000, 0.000000000000000000, -1.000000000000000000 ) ) ;
#5764=LINE ( 'NONE', #1796, #14565 ) ;
#5777=FACE_OUTER_BOUND ( 'NONE', #8983, .T. ) ;
#5789=DIRECTION ( 'NONE',  ( -0.000000000000000000, -1.000000000000000000, -0.000000000000000000 ) ) ;
#5820=CARTESIAN_POINT ( 'NONE',  ( 12.00000000000000000, 0.000000000000000000, -1.469576158976823947E-15 ) ) ;
#5826=DIRECTION ( 'NONE',  ( -1.000000000000000000, -4.625929269271486900E-16, 1.224646799147353207E-16 ) ) ;
#5854=CARTESIAN_POINT ( 'NONE',  ( 27.50000000000000000, 4.500000000000006217, -36.31025403784446581 ) ) ;
#5861=DIRECTION ( 'NONE',  ( 0.000000000000000000, -1.000000000000000000, 0.000000000000000000 ) ) ;
#5868=DIRECTION ( 'NONE',  ( 0.000000000000000000, 0.000000000000000000, 1.000000000000000000 ) ) ;
#5892=ADVANCED_BREP_SHAPE_REPRESENTATION ( '', ( #6561, #7318 ), #21755 ) ;
#5896=EDGE_CURVE ( 'NONE', #13541, #1913, #690, .T. ) ;
#5914=VERTEX_POINT ( 'NONE', #13651 ) ;
#5917=CIRCLE ( 'NONE', #23496, 2.500000000000000444 ) ;
#5919=VERTEX_POINT ( 'NONE', #1159 ) ;
#5949=CARTESIAN_POINT ( 'NONE',  ( 60.00000000000000000, 9.999999999999998224, 17.49999999999999645 ) ) ;
#5960=AXIS2_PLACEMENT_3D ( 'NONE', #4296, #17357, #17476 ) ;
#5967=DIRECTION ( 'NONE',  ( 0.000000000000000000, -1.000000000000000000, 0.000000000000000000 ) ) ;
#5973=ADVANCED_FACE ( 'NONE', ( #6215, #15457 ), #22967, .F. ) ;
#5985=DIRECTION ( 'NONE',  ( 1.000000000000000000, 0.000000000000000000, -0.000000000000000000 ) ) ;
#6020=ADVANCED_FACE ( 'NONE', ( #6803, #23558, #14123 ), #21387, .F. ) ;
#6040=DIRECTION ( 'NONE',  ( -1.000000000000000000, 0.000000000000000000, 0.000000000000000000 ) ) ;
#6059=ORIENTED_EDGE ( 'NONE', *, *, #5699, .T. ) ;
#6078=VECTOR ( 'NONE', #20419, 1000.000000000000000 ) ;
#6137=EDGE_CURVE ( 'NONE', #9090, #7429, #1633, .T. ) ;
#6154=CARTESIAN_POINT ( 'NONE',  ( 19.99999999999999645, 4.500000000000003553, -50.00000000000000000 ) ) ;
#6172=DIRECTION ( 'NONE',  ( 1.000000000000000000, 0.000000000000000000, -1.224646799147353207E-16 ) ) ;
#6175=DIRECTION ( 'NONE',  ( -0.000000000000000000, -0.000000000000000000, 1.000000000000000000 ) ) ;
#6177=DIRECTION ( 'NONE',  ( 1.000000000000000000, -0.000000000000000000, -0.000000000000000000 ) ) ;
#6195=VERTEX_POINT ( 'NONE', #19835 ) ;
#6198=EDGE_CURVE ( 'NONE', #14695, #5303, #11124, .T. ) ;
#6202=ORIENTED_EDGE ( 'NONE', *, *, #7337, .F. ) ;
#6210=CARTESIAN_POINT ( 'NONE',  ( -54.99999999999992895, 15.00000000000000000, 1.387778780781445676E-14 ) ) ;
#6215=FACE_BOUND ( 'NONE', #2902, .T. ) ;
#6241=CARTESIAN_POINT ( 'NONE',  ( -65.00000000000000000, 15.00000000000000000, 10.00000000000008882 ) ) ;
#6245=ORIENTED_EDGE ( 'NONE', *, *, #7610, .T. ) ;
#6260=FACE_OUTER_BOUND ( 'NONE', #7015, .T. ) ;
#6263=EDGE_CURVE ( 'NONE', #8909, #660, #13153, .T. ) ;
#6273=ORIENTED_EDGE ( 'NONE', *, *, #1462, .F. ) ;
#6279=ORIENTED_EDGE ( 'NONE', *, *, #1739, .T. ) ;
#6289=ADVANCED_FACE ( 'NONE', ( #13040 ), #7759, .F. ) ;
#6306=SHAPE_REPRESENTATION_RELATIONSHIP ( 'NONE' , 'NONE' ,  #13579, #5892 ) ;
#6334=ADVANCED_FACE ( 'NONE', ( #22941, #11607, #10045 ), #23054, .T. ) ;
#6337=DIRECTION ( 'NONE',  ( -1.000000000000000000, 0.000000000000000000, 1.224646799147353207E-16 ) ) ;
#6339=CIRCLE ( 'NONE', #18956, 5.000000000000000888 ) ;
#6353=DIRECTION ( 'NONE',  ( 0.000000000000000000, 0.000000000000000000, -1.000000000000000000 ) ) ;
#6354=AXIS2_PLACEMENT_3D ( 'NONE', #12799, #12330, #16372 ) ;
#6359=DIRECTION ( 'NONE',  ( 0.000000000000000000, 0.000000000000000000, -1.000000000000000000 ) ) ;
#6373=ORIENTED_EDGE ( 'NONE', *, *, #13376, .F. ) ;
#6374=VERTEX_POINT ( 'NONE', #4270 ) ;
#6384=CARTESIAN_POINT ( 'NONE',  ( -35.00000000000000711, 4.500000000000003553, -49.99999999999999289 ) ) ;
#6393=VERTEX_POINT ( 'NONE', #20888 ) ;
#6403=VECTOR ( 'NONE', #1431, 1000.000000000000000 ) ;
#6430=VERTEX_POINT ( 'NONE', #1133 ) ;
#6443=FACE_OUTER_BOUND ( 'NONE', #9114, .T. ) ;
#6458=DIRECTION ( 'NONE',  ( -1.000000000000000000, 0.000000000000000000, 1.224646799147352961E-16 ) ) ;
#6461=ORIENTED_EDGE ( 'NONE', *, *, #16570, .F. ) ;
#6462=CIRCLE ( 'NONE', #16039, 4.999999999999997335 ) ;
#6471=ORIENTED_EDGE ( 'NONE', *, *, #18420, .F. ) ;
#6474=CIRCLE ( 'NONE', #1475, 5.000000000000000888 ) ;
#6514=AXIS2_PLACEMENT_3D ( 'NONE', #7220, #9143, #14412 ) ;
#6552=ORIENTED_EDGE ( 'NONE', *, *, #11023, .T. ) ;
#6561=MANIFOLD_SOLID_BREP ( 'M5 Clearance Hole1', #8969 ) ;
#6571=EDGE_CURVE ( 'NONE', #2236, #12336, #16748, .T. ) ;
#6572=DIRECTION ( 'NONE',  ( -0.000000000000000000, -0.000000000000000000, 1.000000000000000000 ) ) ;
#6575=CARTESIAN_POINT ( 'NONE',  ( -60.00000000000000711, 15.00000000000000000, 25.00000000000001421 ) ) ;
#6590=CARTESIAN_POINT ( 'NONE',  ( 19.99999999999999645, 16.40063509461079860, -43.12916512459904084 ) ) ;
#6601=VERTEX_POINT ( 'NONE', #1722 ) ;
#6627=ORIENTED_EDGE ( 'NONE', *, *, #17184, .F. ) ;
#6636=EDGE_CURVE ( 'NONE', #4939, #2701, #20278, .T. ) ;
#6644=FACE_OUTER_BOUND ( 'NONE', #12367, .T. ) ;
#6658=ORIENTED_EDGE ( 'NONE', *, *, #18404, .F. ) ;
#6688=CARTESIAN_POINT ( 'NONE',  ( 60.00000000000000000, -10.00000000000000178, 17.49999999999999645 ) ) ;
#6693=CIRCLE ( 'NONE', #16641, 5.000000000000004441 ) ;
#6719=CARTESIAN_POINT ( 'NONE',  ( -4.898587196589412829E-16, 0.000000000000000000, -4.000000000000000000 ) ) ;
#6767=CARTESIAN_POINT ( 'NONE',  ( -60.00000000000000711, -10.00000000000000178, 12.49999999999999467 ) ) ;
#6769=CARTESIAN_POINT ( 'NONE',  ( 55.00000000000000711, -15.00000000000000000, 19.99999999999999645 ) ) ;
#6775=ORIENTED_EDGE ( 'NONE', *, *, #22976, .T. ) ;
#6777=CARTESIAN_POINT ( 'NONE',  ( 0.000000000000000000, 0.000000000000000000, 0.000000000000000000 ) ) ;
#6793=LINE ( 'NONE', #21025, #4012 ) ;
#6796=ORIENTED_EDGE ( 'NONE', *, *, #9994, .T. ) ;
#6799=DIRECTION ( 'NONE',  ( 0.000000000000000000, 0.000000000000000000, 1.000000000000000000 ) ) ;
#6800=COLOUR_RGB ( '', 0.66274510, 0.83137255, 0.94901961) ;
#6802=ORIENTED_EDGE ( 'NONE', *, *, #12223, .F. ) ;
#6803=FACE_BOUND ( 'NONE', #3252, .T. ) ;
#6825=FILL_AREA_STYLE ('',( #23215 ) ) ;
#6828=EDGE_CURVE ( 'NONE', #13267, #3743, #16946, .T. ) ;
#6882=DIRECTION ( 'NONE',  ( 1.000000000000000000, -0.000000000000000000, -0.000000000000000000 ) ) ;
#6903=ORIENTED_EDGE ( 'NONE', *, *, #1730, .F. ) ;
#6968=CYLINDRICAL_SURFACE ( 'NONE', #18627, 5.000000000000000888 ) ;
#6971=CARTESIAN_POINT ( 'NONE',  ( -65.00000000000000000, -10.00000000000000178, 17.49999999999999645 ) ) ;
#6972=FACE_OUTER_BOUND ( 'NONE', #14656, .T. ) ;
#7003=CARTESIAN_POINT ( 'NONE',  ( -12.00000000000000000, 1.469576158976823947E-15, 1.469576158976823947E-15 ) ) ;
#7015=EDGE_LOOP ( 'NONE', ( #23088, #10189, #16447, #3464 ) ) ;
#7018=( NAMED_UNIT ( * ) SI_UNIT ( $, .STERADIAN. ) SOLID_ANGLE_UNIT ( ) );
#7021=FACE_BOUND ( 'NONE', #21632, .T. ) ;
#7045=DIRECTION ( 'NONE',  ( 1.000000000000000000, 0.000000000000000000, -0.000000000000000000 ) ) ;
#7080=FACE_OUTER_BOUND ( 'NONE', #23387, .T. ) ;
#7101=VERTEX_POINT ( 'NONE', #4710 ) ;
#7131=DIRECTION ( 'NONE',  ( 1.000000000000000000, -0.000000000000000000, -0.000000000000000000 ) ) ;
#7140=( NAMED_UNIT ( * ) PLANE_ANGLE_UNIT ( ) SI_UNIT ( $, .RADIAN. ) );
#7143=ORIENTED_EDGE ( 'NONE', *, *, #15201, .F. ) ;
#7157=CARTESIAN_POINT ( 'NONE',  ( 65.00000000000000000, -9.999999999999998224, 24.99999999999999645 ) ) ;
#7164=EDGE_CURVE ( 'NONE', #12363, #19458, #20214, .T. ) ;
#7181=ORIENTED_EDGE ( 'NONE', *, *, #11967, .F. ) ;
#7209=EDGE_CURVE ( 'NONE', #12336, #2236, #8334, .T. ) ;
#7212=EDGE_CURVE ( 'NONE', #16384, #19904, #13706, .T. ) ;
#7220=CARTESIAN_POINT ( 'NONE',  ( -27.50000000000000711, 4.500000000000003553, -33.66025403784446723 ) ) ;
#7224=DIRECTION ( 'NONE',  ( 0.000000000000000000, 0.000000000000000000, -1.000000000000000000 ) ) ;
#7256=ORIENTED_EDGE ( 'NONE', *, *, #17184, .T. ) ;
#7268=ORIENTED_EDGE ( 'NONE', *, *, #16511, .F. ) ;
#7284=CARTESIAN_POINT ( 'NONE',  ( 35.00000000000000000, 4.500000000000009770, -4.286263797015736496E-15 ) ) ;
#7295=EDGE_LOOP ( 'NONE', ( #19397, #22480, #20882, #5603, #17634 ) ) ;
#7318=AXIS2_PLACEMENT_3D ( 'NONE', #3111, #10686, #17843 ) ;
#7331=FACE_OUTER_BOUND ( 'NONE', #23174, .T. ) ;
#7337=EDGE_CURVE ( 'NONE', #10020, #6374, #22614, .T. ) ;
#7350=EDGE_CURVE ( 'NONE', #1924, #2020, #12575, .T. ) ;
#7368=CARTESIAN_POINT ( 'NONE',  ( 65.00000000000000000, 9.999999999999998224, 14.99999999999999645 ) ) ;
#7373=CARTESIAN_POINT ( 'NONE',  ( 60.00000000000000000, -10.00000000000000178, 12.49999999999999467 ) ) ;
#7386=CARTESIAN_POINT ( 'NONE',  ( -54.99999999999992895, -15.00000000000000000, 1.387778780781445676E-14 ) ) ;
#7405=ORIENTED_EDGE ( 'NONE', *, *, #6198, .F. ) ;
#7429=VERTEX_POINT ( 'NONE', #17359 ) ;
#7500=CYLINDRICAL_SURFACE ( 'NONE', #17494, 9.999999999999996447 ) ;
#7508=DIRECTION ( 'NONE',  ( 1.000000000000000000, 0.000000000000000000, 0.000000000000000000 ) ) ;
#7534=CARTESIAN_POINT ( 'NONE',  ( 55.00000000000000711, 15.00000000000000000, 10.00000000000000000 ) ) ;
#7538=DIRECTION ( 'NONE',  ( 6.123233995736706871E-17, 0.8660254037844414832, 0.4999999999999951705 ) ) ;
#7547=FACE_BOUND ( 'NONE', #731, .T. ) ;
#7561=EDGE_LOOP ( 'NONE', ( #21811, #7181 ) ) ;
#7610=EDGE_CURVE ( 'NONE', #8473, #589, #2704, .T. ) ;
#7614=AXIS2_PLACEMENT_3D ( 'NONE', #17363, #19257, #20919 ) ;
#7642=ADVANCED_FACE ( 'NONE', ( #548 ), #15435, .T. ) ;
#7650=AXIS2_PLACEMENT_3D ( 'NONE', #1284, #937, #6353 ) ;
#7665=VERTEX_POINT ( 'NONE', #5949 ) ;
#7673=EDGE_CURVE ( 'NONE', #12363, #7665, #23635, .T. ) ;
#7709=PLANE ( 'NONE',  #197 ) ;
#7711=AXIS2_PLACEMENT_3D ( 'NONE', #9337, #3570, #18417 ) ;
#7729=CARTESIAN_POINT ( 'NONE',  ( 19.99999999999999645, 1.500000000000003109, -50.00000000000000000 ) ) ;
#7759=CYLINDRICAL_SURFACE ( 'NONE', #15987, 2.649999999999999467 ) ;
#7771=ORIENTED_EDGE ( 'NONE', *, *, #18420, .T. ) ;
#7819=ORIENTED_EDGE ( 'NONE', *, *, #7209, .T. ) ;
#7820=FACE_OUTER_BOUND ( 'NONE', #7295, .T. ) ;
#7822=ORIENTED_EDGE ( 'NONE', *, *, #6263, .F. ) ;
#7841=CARTESIAN_POINT ( 'NONE',  ( 65.00000000000000000, 9.999999999999998224, 19.99999999999999645 ) ) ;
#7846=VECTOR ( 'NONE', #2974, 1000.000000000000000 ) ;
#7855=DIRECTION ( 'NONE',  ( 1.000000000000000000, -0.000000000000000000, -0.000000000000000000 ) ) ;
#7872=DIRECTION ( 'NONE',  ( 1.000000000000000000, -0.000000000000000000, -0.000000000000000000 ) ) ;
#7881=ORIENTED_EDGE ( 'NONE', *, *, #10537, .T. ) ;
#7888=LINE ( 'NONE', #11620, #21211 ) ;
#7902=DIRECTION ( 'NONE',  ( 1.000000000000000000, 4.625929269271485914E-16, -1.224646799147353454E-16 ) ) ;
#7937=VERTEX_POINT ( 'NONE', #7386 ) ;
#7976=CARTESIAN_POINT ( 'NONE',  ( 60.00000000000000711, 15.00000000000000000, 10.00000000000007105 ) ) ;
#7979=DIRECTION ( 'NONE',  ( 1.224646799147353207E-16, -0.000000000000000000, 1.000000000000000000 ) ) ;
#8002=AXIS2_PLACEMENT_3D ( 'NONE', #22434, #17193, #771 ) ;
#8086=LINE ( 'NONE', #6154, #15345 ) ;
#8098=ORIENTED_EDGE ( 'NONE', *, *, #1462, .T. ) ;
#8170=EDGE_LOOP ( 'NONE', ( #5027, #11985, #19894, #15942 ) ) ;
#8173=EDGE_LOOP ( 'NONE', ( #22009, #12284, #356, #3382 ) ) ;
#8194=CARTESIAN_POINT ( 'NONE',  ( 60.00000000000000711, 15.00000000000000000, 24.99999999999999645 ) ) ;
#8220=EDGE_CURVE ( 'NONE', #19365, #11955, #8739, .T. ) ;
#8225=LINE ( 'NONE', #8471, #11242 ) ;
#8231=EDGE_CURVE ( 'NONE', #6195, #14695, #766, .T. ) ;
#8237=ORIENTED_EDGE ( 'NONE', *, *, #20338, .T. ) ;
#8246=CARTESIAN_POINT ( 'NONE',  ( -60.00000000000000711, 15.00000000000000000, 10.00000000000008882 ) ) ;
#8248=CARTESIAN_POINT ( 'NONE',  ( 55.00000000000000711, -9.999999999999998224, 19.99999999999999645 ) ) ;
#8253=DIRECTION ( 'NONE',  ( 0.000000000000000000, 0.000000000000000000, -1.000000000000000000 ) ) ;
#8274=ORIENTED_EDGE ( 'NONE', *, *, #17745, .T. ) ;
#8276=CARTESIAN_POINT ( 'NONE',  ( -4.898587196589412829E-16, 0.000000000000000000, -4.000000000000000000 ) ) ;
#8277=CARTESIAN_POINT ( 'NONE',  ( -65.00000000000000000, -10.00000000000000178, 14.99999999999999467 ) ) ;
#8293=ORIENTED_EDGE ( 'NONE', *, *, #11967, .T. ) ;
#8296=CARTESIAN_POINT ( 'NONE',  ( -35.00000000000000000, 1.500000000000003109, -17.32050807568893092 ) ) ;
#8302=CARTESIAN_POINT ( 'NONE',  ( 9.000000000000000000, 0.000000000000000000, -1.102182119232617714E-15 ) ) ;
#8304=LINE ( 'NONE', #6384, #18512 ) ;
#8334=CIRCLE ( 'NONE', #288, 12.00000000000000000 ) ;
#8335=DIRECTION ( 'NONE',  ( 1.000000000000000000, -0.000000000000000000, -1.224646799147353454E-16 ) ) ;
#8376=DIRECTION ( 'NONE',  ( -1.000000000000000000, 0.000000000000000000, 1.239088197126290817E-16 ) ) ;
#8379=DIRECTION ( 'NONE',  ( 0.000000000000000000, 0.000000000000000000, 1.000000000000000000 ) ) ;
#8384=AXIS2_PLACEMENT_3D ( 'NONE', #15235, #18805, #2271 ) ;
#8394=FACE_OUTER_BOUND ( 'NONE', #10219, .T. ) ;
#8396=ADVANCED_FACE ( 'NONE', ( #12285 ), #10952, .F. ) ;
#8401=AXIS2_PLACEMENT_3D ( 'NONE', #14137, #21403, #22858 ) ;
#8413=LINE ( 'NONE', #19626, #23138 ) ;
#8416=VECTOR ( 'NONE', #1320, 1000.000000000000000 ) ;
#8428=AXIS2_PLACEMENT_3D ( 'NONE', #5196, #14568, #19563 ) ;
#8439=CIRCLE ( 'NONE', #9585, 12.00000000000000000 ) ;
#8440=ORIENTED_EDGE ( 'NONE', *, *, #3399, .F. ) ;
#8471=CARTESIAN_POINT ( 'NONE',  ( -60.00000000000000711, 15.00000000000000000, 10.00000000000004974 ) ) ;
#8473=VERTEX_POINT ( 'NONE', #11192 ) ;
#8484=EDGE_CURVE ( 'NONE', #5362, #1913, #19784, .T. ) ;
#8499=ADVANCED_FACE ( 'NONE', ( #16330 ), #1694, .F. ) ;
#8515=CARTESIAN_POINT ( 'NONE',  ( -54.99999999999992895, 15.00000000000000000, 1.387778780781445676E-14 ) ) ;
#8530=EDGE_CURVE ( 'NONE', #17536, #9561, #12646, .T. ) ;
#8583=ORIENTED_EDGE ( 'NONE', *, *, #18724, .F. ) ;
#8595=FACE_OUTER_BOUND ( 'NONE', #18849, .T. ) ;
#8600=LINE ( 'NONE', #21499, #13245 ) ;
#8604=CARTESIAN_POINT ( 'NONE',  ( -20.00000000000001066, 16.40063509461079150, -43.12916512459904084 ) ) ;
#8624=LINE ( 'NONE', #6590, #1099 ) ;
#8631=CARTESIAN_POINT ( 'NONE',  ( -35.00000000000000000, -8.499999999999966249, 1.285879139104720791E-14 ) ) ;
#8633=AXIS2_PLACEMENT_3D ( 'NONE', #11711, #296, #20657 ) ;
#8636=ORIENTED_EDGE ( 'NONE', *, *, #18431, .T. ) ;
#8643=DIRECTION ( 'NONE',  ( -0.000000000000000000, -0.000000000000000000, 1.000000000000000000 ) ) ;
#8681=DIRECTION ( 'NONE',  ( 1.000000000000000000, 0.000000000000000000, -4.093947403305266636E-14 ) ) ;
#8694=DIRECTION ( 'NONE',  ( -0.000000000000000000, -1.000000000000000000, 0.000000000000000000 ) ) ;
#8739=CIRCLE ( 'NONE', #20177, 9.000000000000000000 ) ;
#8772=LINE ( 'NONE', #19759, #14453 ) ;
#8775=CARTESIAN_POINT ( 'NONE',  ( -65.00000000000000000, -9.999999999999998224, 20.00000000000001421 ) ) ;
#8791=ADVANCED_FACE ( 'NONE', ( #10871 ), #7500, .T. ) ;
#8799=ORIENTED_EDGE ( 'NONE', *, *, #13381, .F. ) ;
#8806=EDGE_CURVE ( 'NONE', #4502, #19518, #11100, .T. ) ;
#8825=VECTOR ( 'NONE', #10236, 1000.000000000000000 ) ;
#8850=DIRECTION ( 'NONE',  ( 0.000000000000000000, -1.000000000000000000, 0.000000000000000000 ) ) ;
#8903=LINE ( 'NONE', #14540, #4689 ) ;
#8909=VERTEX_POINT ( 'NONE', #8296 ) ;
#8918=CIRCLE ( 'NONE', #21488, 7.000000000000000000 ) ;
#8920=ORIENTED_EDGE ( 'NONE', *, *, #7164, .F. ) ;
#8969=CLOSED_SHELL ( 'NONE', ( #6289, #1675, #1582, #14220, #14231, #416, #11540, #14640, #19845, #22597, #19912, #3561, #6020, #12321, #22045, #8791, #7642, #6334, #20504, #16103, #21951, #5973, #10168, #2141, #16925, #11251, #10699, #10264, #1569, #5429, #5117, #10677, #10984, #8396, #21026, #17577, #21956, #5254, #13968, #12218, #17310, #22497, #13479, #20499, #15672, #3800, #15169, #17477, #9073, #8499 ) ) ;
#8974=CARTESIAN_POINT ( 'NONE',  ( 20.00000000000000000, 1.500000000000003109, -17.32050807568893092 ) ) ;
#8981=VERTEX_POINT ( 'NONE', #21667 ) ;
#8983=EDGE_LOOP ( 'NONE', ( #6279, #10372, #13076, #8636 ) ) ;
#9005=ORIENTED_EDGE ( 'NONE', *, *, #12635, .F. ) ;
#9011=ORIENTED_EDGE ( 'NONE', *, *, #3034, .T. ) ;
#9023=PLANE ( 'NONE',  #3616 ) ;
#9035=ORIENTED_EDGE ( 'NONE', *, *, #91, .F. ) ;
#9037=ORIENTED_EDGE ( 'NONE', *, *, #1471, .T. ) ;
#9038=CIRCLE ( 'NONE', #6354, 5.000000000000000888 ) ;
#9042=CIRCLE ( 'NONE', #16046, 5.000000000000000888 ) ;
#9054=DIRECTION ( 'NONE',  ( 0.000000000000000000, 0.000000000000000000, -1.000000000000000000 ) ) ;
#9073=ADVANCED_FACE ( 'NONE', ( #21791 ), #18326, .F. ) ;
#9075=CARTESIAN_POINT ( 'NONE',  ( 27.50000000000000000, 4.500000000000006217, -31.01025403784446510 ) ) ;
#9083=FACE_OUTER_BOUND ( 'NONE', #17969, .T. ) ;
#9090=VERTEX_POINT ( 'NONE', #18209 ) ;
#9099=DIRECTION ( 'NONE',  ( 0.000000000000000000, 0.000000000000000000, 1.000000000000000000 ) ) ;
#9101=ORIENTED_EDGE ( 'NONE', *, *, #8530, .F. ) ;
#9114=EDGE_LOOP ( 'NONE', ( #16850, #13570, #10044, #3663 ) ) ;
#9139=CIRCLE ( 'NONE', #12199, 2.500000000000002220 ) ;
#9143=DIRECTION ( 'NONE',  ( -0.000000000000000000, -1.000000000000000000, 0.000000000000000000 ) ) ;
#9167=VECTOR ( 'NONE', #20332, 1000.000000000000000 ) ;
#9171=DIRECTION ( 'NONE',  ( 0.000000000000000000, 0.000000000000000000, -1.000000000000000000 ) ) ;
#9176=FACE_OUTER_BOUND ( 'NONE', #19687, .T. ) ;
#9189=AXIS2_PLACEMENT_3D ( 'NONE', #21601, #23532, #12786 ) ;
#9192=DIRECTION ( 'NONE',  ( -0.000000000000000000, -1.000000000000000000, -0.000000000000000000 ) ) ;
#9207=DIRECTION ( 'NONE',  ( -4.625929269271486900E-16, 1.000000000000000000, 5.665129472695380173E-32 ) ) ;
#9208=CARTESIAN_POINT ( 'NONE',  ( -65.00000000000000000, -10.00000000000000178, 14.99999999999999467 ) ) ;
#9211=AXIS2_PLACEMENT_3D ( 'NONE', #12405, #19670, #10618 ) ;
#9213=ORIENTED_EDGE ( 'NONE', *, *, #12262, .F. ) ;
#9218=ORIENTED_EDGE ( 'NONE', *, *, #15566, .T. ) ;
#9232=EDGE_CURVE ( 'NONE', #21915, #18272, #23696, .T. ) ;
#9236=EDGE_CURVE ( 'NONE', #22617, #21471, #1498, .T. ) ;
#9272=DIRECTION ( 'NONE',  ( 1.000000000000000000, 0.000000000000000000, -0.000000000000000000 ) ) ;
#9273=ORIENTED_EDGE ( 'NONE', *, *, #23233, .F. ) ;
#9287=ORIENTED_EDGE ( 'NONE', *, *, #17805, .F. ) ;
#9296=DIRECTION ( 'NONE',  ( 1.000000000000000000, -0.000000000000000000, -0.000000000000000000 ) ) ;
#9314=CARTESIAN_POINT ( 'NONE',  ( 65.00000000000000000, -15.00000000000000000, 10.00000000000007105 ) ) ;
#9315=CARTESIAN_POINT ( 'NONE',  ( -60.00000000000000711, 15.00000000000000000, 10.00000000000004974 ) ) ;
#9332=PRODUCT_DEFINITION_SHAPE ( 'NONE', 'NONE',  #18958 ) ;
#9337=CARTESIAN_POINT ( 'NONE',  ( -65.00000000000000000, 9.999999999999998224, 14.99999999999999645 ) ) ;
#9438=ORIENTED_EDGE ( 'NONE', *, *, #18724, .T. ) ;
#9482=DIRECTION ( 'NONE',  ( -0.000000000000000000, 1.000000000000000000, -0.000000000000000000 ) ) ;
#9536=VERTEX_POINT ( 'NONE', #15813 ) ;
#9555=LINE ( 'NONE', #20293, #11517 ) ;
#9561=VERTEX_POINT ( 'NONE', #19726 ) ;
#9566=ORIENTED_EDGE ( 'NONE', *, *, #18490, .F. ) ;
#9585=AXIS2_PLACEMENT_3D ( 'NONE', #235, #14888, #1919 ) ;
#9590=CARTESIAN_POINT ( 'NONE',  ( 54.99999999999992895, 15.00000000000000000, 1.836970198721037478E-15 ) ) ;
#9595=DIRECTION ( 'NONE',  ( -1.000000000000000000, 0.000000000000000000, 0.000000000000000000 ) ) ;
#9654=ORIENTED_EDGE ( 'NONE', *, *, #16388, .T. ) ;
#9685=CARTESIAN_POINT ( 'NONE',  ( -54.99999999999992895, -15.00000000000000000, 5.000000000000015987 ) ) ;
#9693=EDGE_CURVE ( 'NONE', #19458, #13106, #13021, .T. ) ;
#9717=AXIS2_PLACEMENT_3D ( 'NONE', #11702, #6177, #13497 ) ;
#9734=VERTEX_POINT ( 'NONE', #9685 ) ;
#9810=CARTESIAN_POINT ( 'NONE',  ( 34.99999999999999289, 1.500000000000009992, -50.00000000000000711 ) ) ;
#9843=VERTEX_POINT ( 'NONE', #23148 ) ;
#9859=ORIENTED_EDGE ( 'NONE', *, *, #7673, .T. ) ;
#9861=EDGE_CURVE ( 'NONE', #18272, #21915, #3060, .T. ) ;
#9881=ORIENTED_EDGE ( 'NONE', *, *, #7673, .F. ) ;
#9928=ORIENTED_EDGE ( 'NONE', *, *, #16511, .T. ) ;
#9938=AXIS2_PLACEMENT_3D ( 'NONE', #22109, #12935, #18653 ) ;
#9949=EDGE_LOOP ( 'NONE', ( #14034, #16004, #15692, #8920 ) ) ;
#9969=AXIS2_PLACEMENT_3D ( 'NONE', #3776, #9207, #21739 ) ;
#9970=LINE ( 'NONE', #17263, #2467 ) ;
#9971=CYLINDRICAL_SURFACE ( 'NONE', #18399, 2.499999999999998668 ) ;
#9994=EDGE_CURVE ( 'NONE', #22866, #15279, #17232, .T. ) ;
#9998=CARTESIAN_POINT ( 'NONE',  ( 55.00000000000000711, -9.999999999999998224, 20.00000000000001421 ) ) ;
#10004=CARTESIAN_POINT ( 'NONE',  ( 65.00000000000000000, -9.999999999999998224, 24.99999999999999645 ) ) ;
#10020=VERTEX_POINT ( 'NONE', #20374 ) ;
#10035=DIRECTION ( 'NONE',  ( -1.000000000000000000, 0.000000000000000000, 1.224646799147353454E-16 ) ) ;
#10044=ORIENTED_EDGE ( 'NONE', *, *, #15412, .F. ) ;
#10045=FACE_OUTER_BOUND ( 'NONE', #22641, .T. ) ;
#10057=CARTESIAN_POINT ( 'NONE',  ( 65.00000000000000000, 15.00000000000000000, 10.00000000000007105 ) ) ;
#10068=VECTOR ( 'NONE', #21383, 1000.000000000000114 ) ;
#10081=FACE_BOUND ( 'NONE', #17705, .T. ) ;
#10089=CARTESIAN_POINT ( 'NONE',  ( 60.00000000000000711, 15.00000000000000000, 10.00000000000007105 ) ) ;
#10125=VERTEX_POINT ( 'NONE', #11916 ) ;
#10131=EDGE_LOOP ( 'NONE', ( #15604, #11963, #20010, #17928 ) ) ;
#10160=DIRECTION ( 'NONE',  ( -1.000000000000000000, 0.000000000000000000, 0.000000000000000000 ) ) ;
#10168=ADVANCED_FACE ( 'NONE', ( #15621 ), #744, .F. ) ;
#10187=CIRCLE ( 'NONE', #23153, 9.999999999999996447 ) ;
#10189=ORIENTED_EDGE ( 'NONE', *, *, #8484, .F. ) ;
#10210=DIRECTION ( 'NONE',  ( 0.000000000000000000, -1.000000000000000000, -0.000000000000000000 ) ) ;
#10219=EDGE_LOOP ( 'NONE', ( #19269, #22939, #693, #17759 ) ) ;
#10220=EDGE_LOOP ( 'NONE', ( #1840, #11555, #9566, #22515 ) ) ;
#10236=DIRECTION ( 'NONE',  ( -0.000000000000000000, -1.000000000000000000, -0.000000000000000000 ) ) ;
#10238=ORIENTED_EDGE ( 'NONE', *, *, #17133, .T. ) ;
#10258=AXIS2_PLACEMENT_3D ( 'NONE', #22698, #10160, #13398 ) ;
#10264=ADVANCED_FACE ( 'NONE', ( #6260 ), #13580, .T. ) ;
#10279=AXIS2_PLACEMENT_3D ( 'NONE', #3353, #8643, #23473 ) ;
#10283=CARTESIAN_POINT ( 'NONE',  ( -65.00000000000000000, -10.00000000000000178, 12.49999999999999467 ) ) ;
#10304=CARTESIAN_POINT ( 'NONE',  ( -65.00000000000000000, -10.00000000000000178, 12.49999999999999467 ) ) ;
#10337=VECTOR ( 'NONE', #2633, 1000.000000000000000 ) ;
#10363=CARTESIAN_POINT ( 'NONE',  ( -9.000000000000000000, 1.102182119232617714E-15, -3.999999999999999112 ) ) ;
#10372=ORIENTED_EDGE ( 'NONE', *, *, #8484, .T. ) ;
#10383=EDGE_CURVE ( 'NONE', #21471, #16245, #23367, .T. ) ;
#10400=EDGE_LOOP ( 'NONE', ( #10601, #9005, #6471, #6627 ) ) ;
#10424=CARTESIAN_POINT ( 'NONE',  ( -60.00000000000000711, -10.00000000000000178, 14.99999999999999467 ) ) ;
#10439=EDGE_CURVE ( 'NONE', #3743, #5362, #6474, .T. ) ;
#10534=DIRECTION ( 'NONE',  ( -1.000000000000000000, 0.000000000000000000, 0.000000000000000000 ) ) ;
#10537=EDGE_CURVE ( 'NONE', #6430, #589, #11174, .T. ) ;
#10539=CARTESIAN_POINT ( 'NONE',  ( -65.00000000000000000, 9.999999999999998224, 17.49999999999999645 ) ) ;
#10576=LINE ( 'NONE', #21656, #17783 ) ;
#10591=DIRECTION ( 'NONE',  ( -1.000000000000000000, 0.000000000000000000, 0.000000000000000000 ) ) ;
#10601=ORIENTED_EDGE ( 'NONE', *, *, #20338, .F. ) ;
#10618=DIRECTION ( 'NONE',  ( 0.000000000000000000, 0.000000000000000000, 1.000000000000000000 ) ) ;
#10626=CARTESIAN_POINT ( 'NONE',  ( 0.000000000000000000, 0.000000000000000000, 1.734723475976807094E-15 ) ) ;
#10635=FILL_AREA_STYLE_COLOUR ( '', #6800 ) ;
#10658=DIRECTION ( 'NONE',  ( -1.224646799147353207E-16, 0.000000000000000000, -1.000000000000000000 ) ) ;
#10672=ORIENTED_EDGE ( 'NONE', *, *, #16855, .F. ) ;
#10676=CARTESIAN_POINT ( 'NONE',  ( 27.50000000000000000, 4.500000000000006217, -33.66025403784446723 ) ) ;
#10677=ADVANCED_FACE ( 'NONE', ( #8394 ), #11764, .F. ) ;
#10686=DIRECTION ( 'NONE',  ( 0.000000000000000000, 0.000000000000000000, 1.000000000000000000 ) ) ;
#10687=ORIENTED_EDGE ( 'NONE', *, *, #4541, .T. ) ;
#10688=AXIS2_PLACEMENT_3D ( 'NONE', #1464, #12291, #3032 ) ;
#10699=ADVANCED_FACE ( 'NONE', ( #17490 ), #2852, .T. ) ;
#10707=CARTESIAN_POINT ( 'NONE',  ( 55.00000000000000711, 15.00000000000000000, 10.00000000000000000 ) ) ;
#10721=AXIS2_PLACEMENT_3D ( 'NONE', #3944, #22136, #5752 ) ;
#10734=DIRECTION ( 'NONE',  ( -1.000000000000000000, 0.000000000000000000, 1.224646799147353207E-16 ) ) ;
#10740=DIRECTION ( 'NONE',  ( 1.000000000000000000, 0.000000000000000000, -9.637352644315595243E-17 ) ) ;
#10743=AXIS2_PLACEMENT_3D ( 'NONE', #8246, #2939, #23178 ) ;
#10760=CYLINDRICAL_SURFACE ( 'NONE', #14536, 9.000000000000000000 ) ;
#10842=EDGE_CURVE ( 'NONE', #5303, #4502, #8624, .T. ) ;
#10865=( LENGTH_UNIT ( ) NAMED_UNIT ( * ) SI_UNIT ( .MILLI., .METRE. ) );
#10871=FACE_OUTER_BOUND ( 'NONE', #22475, .T. ) ;
#10884=CARTESIAN_POINT ( 'NONE',  ( -65.00000000000000000, -9.999999999999998224, 25.00000000000001421 ) ) ;
#10889=EDGE_CURVE ( 'NONE', #19904, #16384, #16423, .T. ) ;
#10894=ORIENTED_EDGE ( 'NONE', *, *, #15921, .T. ) ;
#10918=FACE_OUTER_BOUND ( 'NONE', #18330, .T. ) ;
#10952=CYLINDRICAL_SURFACE ( 'NONE', #15216, 7.000000000000000000 ) ;
#10984=ADVANCED_FACE ( 'NONE', ( #17723 ), #14619, .F. ) ;
#10992=CIRCLE ( 'NONE', #20126, 7.000000000000000000 ) ;
#10996=DIRECTION ( 'NONE',  ( 1.000000000000000000, -0.000000000000000000, -0.000000000000000000 ) ) ;
#10999=ORIENTED_EDGE ( 'NONE', *, *, #16710, .T. ) ;
#11023=EDGE_CURVE ( 'NONE', #19235, #2236, #11143, .T. ) ;
#11025=ORIENTED_EDGE ( 'NONE', *, *, #1873, .F. ) ;
#11069=AXIS2_PLACEMENT_3D ( 'NONE', #8277, #11997, #13795 ) ;
#11081=AXIS2_PLACEMENT_3D ( 'NONE', #22013, #3831, #2017 ) ;
#11097=AXIS2_PLACEMENT_3D ( 'NONE', #16243, #20039, #5566 ) ;
#11100=LINE ( 'NONE', #1962, #3338 ) ;
#11122=ORIENTED_EDGE ( 'NONE', *, *, #18466, .T. ) ;
#11124=LINE ( 'NONE', #3666, #22068 ) ;
#11139=EDGE_LOOP ( 'NONE', ( #19480, #14324 ) ) ;
#11141=CARTESIAN_POINT ( 'NONE',  ( -65.00000000000000000, 9.999999999999998224, 14.99999999999999645 ) ) ;
#11143=LINE ( 'NONE', #20435, #19151 ) ;
#11174=LINE ( 'NONE', #13089, #1866 ) ;
#11192=CARTESIAN_POINT ( 'NONE',  ( -35.00000000000000711, 4.500000000000003553, 1.285879139104720791E-14 ) ) ;
#11217=ORIENTED_EDGE ( 'NONE', *, *, #13381, .T. ) ;
#11232=CARTESIAN_POINT ( 'NONE',  ( 19.99999999999999645, 1.500000000000003109, -50.00000000000000000 ) ) ;
#11234=LINE ( 'NONE', #1630, #941 ) ;
#11235=ORIENTED_EDGE ( 'NONE', *, *, #1873, .T. ) ;
#11242=VECTOR ( 'NONE', #21001, 1000.000000000000000 ) ;
#11251=ADVANCED_FACE ( 'NONE', ( #6443 ), #912, .T. ) ;
#11252=LINE ( 'NONE', #4159, #13001 ) ;
#11266=DIRECTION ( 'NONE',  ( 1.000000000000000000, -0.000000000000000000, -0.000000000000000000 ) ) ;
#11268=PLANE ( 'NONE',  #18537 ) ;
#11341=ORIENTED_EDGE ( 'NONE', *, *, #3688, .T. ) ;
#11361=DIRECTION ( 'NONE',  ( 1.060575238724910366E-16, -0.4999999999999951150, 0.8660254037844414832 ) ) ;
#11383=VECTOR ( 'NONE', #3507, 1000.000000000000000 ) ;
#11389=ORIENTED_EDGE ( 'NONE', *, *, #15921, .F. ) ;
#11395=VECTOR ( 'NONE', #14211, 1000.000000000000000 ) ;
#11440=DIRECTION ( 'NONE',  ( 0.000000000000000000, 0.000000000000000000, 1.000000000000000000 ) ) ;
#11484=DIRECTION ( 'NONE',  ( 1.000000000000000000, -0.000000000000000000, -0.000000000000000000 ) ) ;
#11513=DIRECTION ( 'NONE',  ( -0.000000000000000000, -1.000000000000000000, -0.000000000000000000 ) ) ;
#11517=VECTOR ( 'NONE', #14598, 1000.000000000000000 ) ;
#11530=CARTESIAN_POINT ( 'NONE',  ( -65.00000000000000000, -10.00000000000000178, 14.99999999999999467 ) ) ;
#11540=ADVANCED_FACE ( 'NONE', ( #13556 ), #9971, .F. ) ;
#11555=ORIENTED_EDGE ( 'NONE', *, *, #17291, .T. ) ;
#11573=ORIENTED_EDGE ( 'NONE', *, *, #3652, .T. ) ;
#11607=FACE_BOUND ( 'NONE', #11139, .T. ) ;
#11620=CARTESIAN_POINT ( 'NONE',  ( 34.99999999999999289, 4.500000000000009770, -50.00000000000000711 ) ) ;
#11630=ORIENTED_EDGE ( 'NONE', *, *, #21122, .T. ) ;
#11638=ORIENTED_EDGE ( 'NONE', *, *, #15947, .F. ) ;
#11661=ORIENTED_EDGE ( 'NONE', *, *, #1004, .T. ) ;
#11666=VERTEX_POINT ( 'NONE', #16290 ) ;
#11676=CARTESIAN_POINT ( 'NONE',  ( 55.00000000000000711, 15.00000000000000000, 10.00000000000000000 ) ) ;
#11702=CARTESIAN_POINT ( 'NONE',  ( -65.00000000000000000, 9.999999999999998224, 14.99999999999999645 ) ) ;
#11711=CARTESIAN_POINT ( 'NONE',  ( 55.00000000000000711, 15.00000000000000000, 10.00000000000000000 ) ) ;
#11756=CARTESIAN_POINT ( 'NONE',  ( 54.99999999999992895, 15.00000000000000000, 1.836970198721037478E-15 ) ) ;
#11764=CYLINDRICAL_SURFACE ( 'NONE', #11069, 2.499999999999998668 ) ;
#11774=ORIENTED_EDGE ( 'NONE', *, *, #18099, .F. ) ;
#11775=CARTESIAN_POINT ( 'NONE',  ( 65.00000000000000000, 9.999999999999998224, 12.49999999999999289 ) ) ;
#11779=EDGE_LOOP ( 'NONE', ( #1305, #20865, #22401, #3161, #13814 ) ) ;
#11781=ORIENTED_EDGE ( 'NONE', *, *, #15566, .F. ) ;
#11804=CARTESIAN_POINT ( 'NONE',  ( -12.00000000000000000, 1.469576158976823947E-15, -3.999999999999998224 ) ) ;
#11809=ORIENTED_EDGE ( 'NONE', *, *, #18424, .T. ) ;
#11837=VERTEX_POINT ( 'NONE', #4049 ) ;
#11869=DIRECTION ( 'NONE',  ( -1.224646799147353207E-16, 0.000000000000000000, -1.000000000000000000 ) ) ;
#11874=FACE_OUTER_BOUND ( 'NONE', #1979, .T. ) ;
#11910=VECTOR ( 'NONE', #23485, 1000.000000000000000 ) ;
#11916=CARTESIAN_POINT ( 'NONE',  ( 60.00000000000000711, 15.00000000000000000, 19.99999999999999645 ) ) ;
#11929=EDGE_CURVE ( 'NONE', #15611, #7937, #2832, .T. ) ;
#11955=VERTEX_POINT ( 'NONE', #20908 ) ;
#11963=ORIENTED_EDGE ( 'NONE', *, *, #10889, .F. ) ;
#11967=EDGE_CURVE ( 'NONE', #16436, #6393, #12661, .T. ) ;
#11976=ORIENTED_EDGE ( 'NONE', *, *, #15985, .F. ) ;
#11983=AXIS2_PLACEMENT_3D ( 'NONE', #10424, #19359, #6799 ) ;
#11985=ORIENTED_EDGE ( 'NONE', *, *, #10383, .T. ) ;
#11997=DIRECTION ( 'NONE',  ( 1.000000000000000000, -0.000000000000000000, -0.000000000000000000 ) ) ;
#12001=LINE ( 'NONE', #14019, #7846 ) ;
#12020=EDGE_CURVE ( 'NONE', #7665, #12363, #21407, .T. ) ;
#12106=VECTOR ( 'NONE', #103, 1000.000000000000000 ) ;
#12153=DIRECTION ( 'NONE',  ( -0.000000000000000000, 1.000000000000000000, -0.000000000000000000 ) ) ;
#12154=ORIENTED_EDGE ( 'NONE', *, *, #15806, .F. ) ;
#12162=CARTESIAN_POINT ( 'NONE',  ( -60.00000000000000711, 9.999999999999998224, 25.00000000000001421 ) ) ;
#12163=VECTOR ( 'NONE', #23390, 1000.000000000000000 ) ;
#12179=DIRECTION ( 'NONE',  ( 1.000000000000000000, 0.000000000000000000, 0.000000000000000000 ) ) ;
#12199=AXIS2_PLACEMENT_3D ( 'NONE', #7368, #18475, #9171 ) ;
#12215=DIRECTION ( 'NONE',  ( -0.000000000000000000, -1.000000000000000000, -0.000000000000000000 ) ) ;
#12218=ADVANCED_FACE ( 'NONE', ( #14713, #9083 ), #69, .F. ) ;
#12223=EDGE_CURVE ( 'NONE', #17685, #1297, #12910, .T. ) ;
#12240=AXIS2_PLACEMENT_3D ( 'NONE', #7534, #5725, #559 ) ;
#12262=EDGE_CURVE ( 'NONE', #3750, #11837, #5351, .T. ) ;
#12271=CARTESIAN_POINT ( 'NONE',  ( 60.00000000000000000, -10.00000000000000178, 14.99999999999999467 ) ) ;
#12284=ORIENTED_EDGE ( 'NONE', *, *, #21059, .F. ) ;
#12285=FACE_OUTER_BOUND ( 'NONE', #22273, .T. ) ;
#12290=EDGE_CURVE ( 'NONE', #15019, #2372, #9555, .T. ) ;
#12291=DIRECTION ( 'NONE',  ( -3.393848863725434895E-16, 0.8660254037844414832, 0.4999999999999951705 ) ) ;
#12321=ADVANCED_FACE ( 'NONE', ( #13148 ), #12801, .T. ) ;
#12330=DIRECTION ( 'NONE',  ( -1.000000000000000000, 0.000000000000000000, 0.000000000000000000 ) ) ;
#12334=LINE ( 'NONE', #18274, #2884 ) ;
#12336=VERTEX_POINT ( 'NONE', #5820 ) ;
#12355=DIRECTION ( 'NONE',  ( -1.000000000000000000, 0.000000000000000000, 0.000000000000000000 ) ) ;
#12362=SURFACE_STYLE_FILL_AREA ( #6825 ) ;
#12363=VERTEX_POINT ( 'NONE', #4492 ) ;
#12367=EDGE_LOOP ( 'NONE', ( #3962, #2100, #16732, #21391, #7881 ) ) ;
#12405=CARTESIAN_POINT ( 'NONE',  ( -65.00000000000000000, -10.00000000000000178, 14.99999999999999467 ) ) ;
#12412=ORIENTED_EDGE ( 'NONE', *, *, #547, .T. ) ;
#12423=DIRECTION ( 'NONE',  ( -1.000000000000000000, 0.000000000000000000, 1.224646799147353207E-16 ) ) ;
#12441=LINE ( 'NONE', #3188, #14388 ) ;
#12444=FACE_BOUND ( 'NONE', #15563, .T. ) ;
#12448=CARTESIAN_POINT ( 'NONE',  ( -60.00000000000000711, 15.00000000000000000, 20.00000000000001421 ) ) ;
#12458=AXIS2_PLACEMENT_3D ( 'NONE', #12726, #11266, #16410 ) ;
#12508=LINE ( 'NONE', #21436, #11910 ) ;
#12521=CARTESIAN_POINT ( 'NONE',  ( 0.000000000000000000, 0.000000000000000000, 1.734723475976807094E-15 ) ) ;
#12522=ORIENTED_EDGE ( 'NONE', *, *, #23233, .T. ) ;
#12532=FACE_OUTER_BOUND ( 'NONE', #954, .T. ) ;
#12537=AXIS2_PLACEMENT_3D ( 'NONE', #20122, #18118, #1813 ) ;
#12549=FILL_AREA_STYLE ('',( #10635 ) ) ;
#12568=AXIS2_PLACEMENT_3D ( 'NONE', #19848, #16391, #20074 ) ;
#12572=CARTESIAN_POINT ( 'NONE',  ( 19.99999999999999645, 4.500000000000003553, -50.00000000000000000 ) ) ;
#12575=CIRCLE ( 'NONE', #2203, 9.000000000000000000 ) ;
#12588=ORIENTED_EDGE ( 'NONE', *, *, #15956, .F. ) ;
#12613=DIRECTION ( 'NONE',  ( 1.224646799147353207E-16, -0.000000000000000000, 1.000000000000000000 ) ) ;
#12627=CARTESIAN_POINT ( 'NONE',  ( 60.00000000000000711, -15.00000000000000000, 10.00000000000007105 ) ) ;
#12635=EDGE_CURVE ( 'NONE', #10125, #1357, #1081, .T. ) ;
#12646=LINE ( 'NONE', #3728, #11383 ) ;
#12661=CIRCLE ( 'NONE', #20650, 2.649999999999999467 ) ;
#12693=DIRECTION ( 'NONE',  ( 1.000000000000000000, -0.000000000000000000, -0.000000000000000000 ) ) ;
#12720=ORIENTED_EDGE ( 'NONE', *, *, #4832, .T. ) ;
#12726=CARTESIAN_POINT ( 'NONE',  ( -65.00000000000000000, -10.00000000000000178, 14.99999999999999467 ) ) ;
#12739=CARTESIAN_POINT ( 'NONE',  ( -60.00000000000000711, 9.999999999999998224, 20.00000000000001421 ) ) ;
#12758=ORIENTED_EDGE ( 'NONE', *, *, #15576, .T. ) ;
#12786=DIRECTION ( 'NONE',  ( 0.000000000000000000, 0.000000000000000000, -1.000000000000000000 ) ) ;
#12799=CARTESIAN_POINT ( 'NONE',  ( 60.00000000000000711, 9.999999999999998224, 19.99999999999999645 ) ) ;
#12801=PLANE ( 'NONE',  #21795 ) ;
#12824=FACE_OUTER_BOUND ( 'NONE', #13717, .T. ) ;
#12846=AXIS2_PLACEMENT_3D ( 'NONE', #329, #13290, #677 ) ;
#12856=APPLICATION_CONTEXT ( 'automotive_design' ) ;
#12859=ORIENTED_EDGE ( 'NONE', *, *, #6828, .T. ) ;
#12869=DIRECTION ( 'NONE',  ( 1.000000000000000000, -0.000000000000000000, -0.000000000000000000 ) ) ;
#12910=LINE ( 'NONE', #11232, #23327 ) ;
#12912=DIRECTION ( 'NONE',  ( -0.000000000000000000, -1.000000000000000000, -0.000000000000000000 ) ) ;
#12935=DIRECTION ( 'NONE',  ( 1.000000000000000000, 0.000000000000000000, 0.000000000000000000 ) ) ;
#12938=VECTOR ( 'NONE', #220, 1000.000000000000000 ) ;
#12949=DIRECTION ( 'NONE',  ( 0.000000000000000000, 0.000000000000000000, -1.000000000000000000 ) ) ;
#12952=ORIENTED_EDGE ( 'NONE', *, *, #17805, .T. ) ;
#12959=VECTOR ( 'NONE', #19084, 1000.000000000000000 ) ;
#12976=EDGE_LOOP ( 'NONE', ( #20354, #14773 ) ) ;
#12977=AXIS2_PLACEMENT_3D ( 'NONE', #15343, #17475, #6337 ) ;
#12989=CIRCLE ( 'NONE', #17940, 9.000000000000000000 ) ;
#13001=VECTOR ( 'NONE', #22232, 1000.000000000000000 ) ;
#13017=ORIENTED_EDGE ( 'NONE', *, *, #3399, .T. ) ;
#13021=CIRCLE ( 'NONE', #3808, 2.500000000000002220 ) ;
#13040=FACE_OUTER_BOUND ( 'NONE', #4825, .T. ) ;
#13062=DIRECTION ( 'NONE',  ( -1.000000000000000000, 0.000000000000000000, 1.224646799147353207E-16 ) ) ;
#13076=ORIENTED_EDGE ( 'NONE', *, *, #5896, .F. ) ;
#13089=CARTESIAN_POINT ( 'NONE',  ( -20.00000000000001066, 4.500000000000003553, -50.00000000000000000 ) ) ;
#13092=FACE_OUTER_BOUND ( 'NONE', #13565, .T. ) ;
#13097=CARTESIAN_POINT ( 'NONE',  ( -7.000000000000000000, 8.572527594031473190E-16, 1.734723475976807094E-15 ) ) ;
#13106=VERTEX_POINT ( 'NONE', #20813 ) ;
#13122=VERTEX_POINT ( 'NONE', #11756 ) ;
#13132=DIRECTION ( 'NONE',  ( -0.000000000000000000, -1.000000000000000000, -0.000000000000000000 ) ) ;
#13148=FACE_OUTER_BOUND ( 'NONE', #14989, .T. ) ;
#13153=LINE ( 'NONE', #20539, #5251 ) ;
#13184=DIRECTION ( 'NONE',  ( -1.000000000000000000, 0.000000000000000000, 1.224646799147353207E-16 ) ) ;
#13189=ORIENTED_EDGE ( 'NONE', *, *, #3034, .F. ) ;
#13212=ORIENTED_EDGE ( 'NONE', *, *, #1201, .T. ) ;
#13217=ORIENTED_EDGE ( 'NONE', *, *, #16570, .T. ) ;
#13227=CIRCLE ( 'NONE', #12846, 2.649999999999999467 ) ;
#13245=VECTOR ( 'NONE', #3434, 1000.000000000000000 ) ;
#13267=VERTEX_POINT ( 'NONE', #5340 ) ;
#13269=CYLINDRICAL_SURFACE ( 'NONE', #22104, 2.499999999999998668 ) ;
#13287=CARTESIAN_POINT ( 'NONE',  ( 27.50000000000000000, 1.500000000000003109, -33.66025403784446723 ) ) ;
#13290=DIRECTION ( 'NONE',  ( -0.000000000000000000, -1.000000000000000000, -0.000000000000000000 ) ) ;
#13293=ORIENTED_EDGE ( 'NONE', *, *, #23465, .T. ) ;
#13318=DIRECTION ( 'NONE',  ( 0.000000000000000000, 0.000000000000000000, -1.000000000000000000 ) ) ;
#13322=CARTESIAN_POINT ( 'NONE',  ( -55.00000000000000000, 15.00000000000000000, 10.00000000000001599 ) ) ;
#13376=EDGE_CURVE ( 'NONE', #17685, #14695, #17192, .T. ) ;
#13381=EDGE_CURVE ( 'NONE', #6601, #18050, #15527, .T. ) ;
#13398=DIRECTION ( 'NONE',  ( 0.000000000000000000, 0.000000000000000000, 1.000000000000000000 ) ) ;
#13421=DIRECTION ( 'NONE',  ( 1.000000000000000000, -0.000000000000000000, -0.000000000000000000 ) ) ;
#13450=CARTESIAN_POINT ( 'NONE',  ( 0.000000000000000000, 0.000000000000000000, 0.000000000000000000 ) ) ;
#13479=ADVANCED_FACE ( 'NONE', ( #6644 ), #5629, .F. ) ;
#13497=DIRECTION ( 'NONE',  ( 0.000000000000000000, 0.000000000000000000, -1.000000000000000000 ) ) ;
#13514=DIRECTION ( 'NONE',  ( 0.000000000000000000, 0.000000000000000000, -1.000000000000000000 ) ) ;
#13523=DIRECTION ( 'NONE',  ( 0.000000000000000000, 0.000000000000000000, 1.000000000000000000 ) ) ;
#13529=LINE ( 'NONE', #19006, #21617 ) ;
#13541=VERTEX_POINT ( 'NONE', #12162 ) ;
#13556=FACE_OUTER_BOUND ( 'NONE', #8170, .T. ) ;
#13565=EDGE_LOOP ( 'NONE', ( #4589, #184, #11389, #7143, #9273, #15186, #9035, #12859, #12758, #12720, #22450, #17265 ) ) ;
#13570=ORIENTED_EDGE ( 'NONE', *, *, #18466, .F. ) ;
#13576=EDGE_CURVE ( 'NONE', #15433, #6393, #18010, .T. ) ;
#13579=SHAPE_REPRESENTATION ( 'Machined Body Housing', ( #7318 ), #21755 ) ;
#13580=CYLINDRICAL_SURFACE ( 'NONE', #15709, 5.000000000000000888 ) ;
#13599=AXIS2_PLACEMENT_3D ( 'NONE', #5136, #21055, #4667 ) ;
#13610=CIRCLE ( 'NONE', #14002, 5.000000000000000888 ) ;
#13642=CARTESIAN_POINT ( 'NONE',  ( -65.00000000000000000, 9.999999999999998224, 12.49999999999999289 ) ) ;
#13651=CARTESIAN_POINT ( 'NONE',  ( 54.99999999999996447, -15.00000000000000000, 5.000000000000003553 ) ) ;
#13653=PRODUCT_DEFINITION_CONTEXT ( 'detailed design', #3495, 'design' ) ;
#13691=CARTESIAN_POINT ( 'NONE',  ( 65.00000000000000000, 15.00000000000000000, 19.99999999999999645 ) ) ;
#13706=CIRCLE ( 'NONE', #21689, 2.649999999999999467 ) ;
#13717=EDGE_LOOP ( 'NONE', ( #16891, #21203, #7822, #22740 ) ) ;
#13754=CIRCLE ( 'NONE', #12240, 9.999999999999996447 ) ;
#13760=CARTESIAN_POINT ( 'NONE',  ( 65.00000000000000000, -10.00000000000000178, 17.49999999999999645 ) ) ;
#13772=AXIS2_PLACEMENT_3D ( 'NONE', #11530, #5985, #5868 ) ;
#13774=VECTOR ( 'NONE', #14979, 1000.000000000000000 ) ;
#13778=DIRECTION ( 'NONE',  ( 1.000000000000000000, -0.000000000000000000, -0.000000000000000000 ) ) ;
#13780=CARTESIAN_POINT ( 'NONE',  ( 19.99999999999999645, 4.500000000000003553, -50.00000000000000000 ) ) ;
#13795=DIRECTION ( 'NONE',  ( 0.000000000000000000, 0.000000000000000000, -1.000000000000000000 ) ) ;
#13799=FACE_OUTER_BOUND ( 'NONE', #11779, .T. ) ;
#13814=ORIENTED_EDGE ( 'NONE', *, *, #10842, .T. ) ;
#13822=COLOUR_RGB ( '', 0.66274510, 0.83137255, 0.94901961) ;
#13842=EDGE_LOOP ( 'NONE', ( #6245, #2872, #4817, #2976 ) ) ;
#13844=EDGE_LOOP ( 'NONE', ( #1750, #18693 ) ) ;
#13848=DIRECTION ( 'NONE',  ( 1.224646799147353207E-16, -0.000000000000000000, 1.000000000000000000 ) ) ;
#13919=ORIENTED_EDGE ( 'NONE', *, *, #15985, .T. ) ;
#13968=ADVANCED_FACE ( 'NONE', ( #17828 ), #21638, .F. ) ;
#14002=AXIS2_PLACEMENT_3D ( 'NONE', #20145, #9296, #2069 ) ;
#14019=CARTESIAN_POINT ( 'NONE',  ( -35.00000000000000711, 1.500000000000003109, -49.99999999999999289 ) ) ;
#14021=ORIENTED_EDGE ( 'NONE', *, *, #9693, .T. ) ;
#14034=ORIENTED_EDGE ( 'NONE', *, *, #12020, .F. ) ;
#14065=ORIENTED_EDGE ( 'NONE', *, *, #17611, .T. ) ;
#14067=AXIS2_PLACEMENT_3D ( 'NONE', #21702, #21462, #19795 ) ;
#14086=CARTESIAN_POINT ( 'NONE',  ( 65.00000000000000000, 9.999999999999998224, 24.99999999999999645 ) ) ;
#14123=FACE_OUTER_BOUND ( 'NONE', #21033, .T. ) ;
#14137=CARTESIAN_POINT ( 'NONE',  ( -20.00000000000001066, 4.500000000000003553, -50.00000000000000000 ) ) ;
#14143=CIRCLE ( 'NONE', #2650, 12.00000000000000000 ) ;
#14160=FACE_OUTER_BOUND ( 'NONE', #15194, .T. ) ;
#14211=DIRECTION ( 'NONE',  ( -1.000000000000000000, 0.000000000000000000, 0.000000000000000000 ) ) ;
#14212=CARTESIAN_POINT ( 'NONE',  ( -35.00000000000000711, 4.500000000000003553, -49.99999999999999289 ) ) ;
#14220=ADVANCED_FACE ( 'NONE', ( #14160 ), #16306, .T. ) ;
#14231=ADVANCED_FACE ( 'NONE', ( #7331 ), #14636, .F. ) ;
#14285=CIRCLE ( 'NONE', #3927, 9.000000000000000000 ) ;
#14324=ORIENTED_EDGE ( 'NONE', *, *, #9861, .T. ) ;
#14327=ORIENTED_EDGE ( 'NONE', *, *, #8220, .T. ) ;
#14351=AXIS2_PLACEMENT_3D ( 'NONE', #19158, #15475, #831 ) ;
#14388=VECTOR ( 'NONE', #17811, 1000.000000000000000 ) ;
#14391=DIRECTION ( 'NONE',  ( 1.000000000000000000, 0.000000000000000000, -1.224646799147353207E-16 ) ) ;
#14395=FACE_BOUND ( 'NONE', #12976, .T. ) ;
#14402=AXIS2_PLACEMENT_3D ( 'NONE', #6719, #21293, #4916 ) ;
#14407=CYLINDRICAL_SURFACE ( 'NONE', #20899, 9.000000000000000000 ) ;
#14412=DIRECTION ( 'NONE',  ( 0.000000000000000000, 0.000000000000000000, -1.000000000000000000 ) ) ;
#14445=LINE ( 'NONE', #14212, #22734 ) ;
#14453=VECTOR ( 'NONE', #23234, 1000.000000000000000 ) ;
#14475=DIRECTION ( 'NONE',  ( -1.000000000000000000, -4.625929269271485914E-16, 1.224646799147353454E-16 ) ) ;
#14478=ORIENTED_EDGE ( 'NONE', *, *, #12020, .T. ) ;
#14536=AXIS2_PLACEMENT_3D ( 'NONE', #1961, #14696, #16476 ) ;
#14540=CARTESIAN_POINT ( 'NONE',  ( -60.00000000000000711, 15.00000000000000000, 10.00000000000008882 ) ) ;
#14542=CARTESIAN_POINT ( 'NONE',  ( 54.99999999999992895, -15.00000000000000000, 5.000000000000001776 ) ) ;
#14555=CARTESIAN_POINT ( 'NONE',  ( -60.00000000000000711, -9.999999999999998224, 25.00000000000001421 ) ) ;
#14564=AXIS2_PLACEMENT_3D ( 'NONE', #16687, #35, #11440 ) ;
#14565=VECTOR ( 'NONE', #9482, 1000.000000000000000 ) ;
#14568=DIRECTION ( 'NONE',  ( 0.000000000000000000, 1.000000000000000000, 0.000000000000000000 ) ) ;
#14581=ORIENTED_EDGE ( 'NONE', *, *, #4603, .F. ) ;
#14596=DIRECTION ( 'NONE',  ( 0.000000000000000000, -1.000000000000000000, -0.000000000000000000 ) ) ;
#14598=DIRECTION ( 'NONE',  ( -1.000000000000000000, 0.000000000000000000, 1.224646799147353454E-16 ) ) ;
#14608=ORIENTED_EDGE ( 'NONE', *, *, #2736, .T. ) ;
#14615=ORIENTED_EDGE ( 'NONE', *, *, #3861, .F. ) ;
#14619=CYLINDRICAL_SURFACE ( 'NONE', #7711, 2.500000000000002220 ) ;
#14632=CARTESIAN_POINT ( 'NONE',  ( -65.00000000000000000, 9.999999999999998224, 20.00000000000001421 ) ) ;
#14636=CYLINDRICAL_SURFACE ( 'NONE', #10279, 7.000000000000000000 ) ;
#14640=ADVANCED_FACE ( 'NONE', ( #11874 ), #697, .F. ) ;
#14656=EDGE_LOOP ( 'NONE', ( #4568, #4857, #2673, #12588, #23129, #19337, #15698, #21042, #10687, #10238, #11217, #792 ) ) ;
#14686=ORIENTED_EDGE ( 'NONE', *, *, #6636, .F. ) ;
#14695=VERTEX_POINT ( 'NONE', #19287 ) ;
#14696=DIRECTION ( 'NONE',  ( 1.224646799147353207E-16, -0.000000000000000000, 1.000000000000000000 ) ) ;
#14713=FACE_BOUND ( 'NONE', #3524, .T. ) ;
#14727=DIRECTION ( 'NONE',  ( 0.000000000000000000, 0.000000000000000000, -1.000000000000000000 ) ) ;
#14751=CARTESIAN_POINT ( 'NONE',  ( -65.00000000000000000, 15.00000000000000000, 10.00000000000008882 ) ) ;
#14762=CARTESIAN_POINT ( 'NONE',  ( -60.00000000000000711, 9.999999999999998224, 17.49999999999999645 ) ) ;
#14773=ORIENTED_EDGE ( 'NONE', *, *, #8220, .F. ) ;
#14784=AXIS2_PLACEMENT_3D ( 'NONE', #5530, #3609, #1930 ) ;
#14796=CARTESIAN_POINT ( 'NONE',  ( -65.00000000000000000, 15.00000000000000000, 25.00000000000001421 ) ) ;
#14815=EDGE_CURVE ( 'NONE', #5234, #16245, #2609, .T. ) ;
#14817=DIRECTION ( 'NONE',  ( -0.000000000000000000, 1.000000000000000000, -0.000000000000000000 ) ) ;
#14851=DIRECTION ( 'NONE',  ( 0.000000000000000000, 0.000000000000000000, -1.000000000000000000 ) ) ;
#14869=CARTESIAN_POINT ( 'NONE',  ( 0.000000000000000000, 0.000000000000000000, 0.000000000000000000 ) ) ;
#14883=ORIENTED_EDGE ( 'NONE', *, *, #10439, .T. ) ;
#14888=DIRECTION ( 'NONE',  ( -1.224646799147353207E-16, 0.000000000000000000, -1.000000000000000000 ) ) ;
#14895=VERTEX_POINT ( 'NONE', #21875 ) ;
#14909=PRODUCT_DEFINITION_FORMATION_WITH_SPECIFIED_SOURCE ( 'ANY', '', #2634, .NOT_KNOWN. ) ;
#14924=EDGE_CURVE ( 'NONE', #11955, #19365, #12989, .T. ) ;
#14934=EDGE_LOOP ( 'NONE', ( #22488, #9881, #23621, #14021 ) ) ;
#14979=DIRECTION ( 'NONE',  ( -0.000000000000000000, -0.000000000000000000, 1.000000000000000000 ) ) ;
#14982=EDGE_CURVE ( 'NONE', #15347, #9734, #2999, .T. ) ;
#14989=EDGE_LOOP ( 'NONE', ( #6775, #11122, #9287, #7256 ) ) ;
#15019=VERTEX_POINT ( 'NONE', #20988 ) ;
#15036=LINE ( 'NONE', #16569, #23061 ) ;
#15096=FACE_OUTER_BOUND ( 'NONE', #20341, .T. ) ;
#15106=EDGE_CURVE ( 'NONE', #4939, #10125, #2329, .T. ) ;
#15168=CARTESIAN_POINT ( 'NONE',  ( 55.00000000000000711, -15.00000000000000000, 20.00000000000001421 ) ) ;
#15169=ADVANCED_FACE ( 'NONE', ( #4719 ), #22918, .F. ) ;
#15172=AXIS2_PLACEMENT_3D ( 'NONE', #22484, #17001, #21036 ) ;
#15186=ORIENTED_EDGE ( 'NONE', *, *, #14982, .F. ) ;
#15193=DIRECTION ( 'NONE',  ( 0.000000000000000000, 0.000000000000000000, -1.000000000000000000 ) ) ;
#15194=EDGE_LOOP ( 'NONE', ( #17608, #6552, #1094, #6273 ) ) ;
#15201=EDGE_CURVE ( 'NONE', #5914, #2701, #6462, .T. ) ;
#15216=AXIS2_PLACEMENT_3D ( 'NONE', #12521, #3612, #21925 ) ;
#15235=CARTESIAN_POINT ( 'NONE',  ( 60.00000000000000711, -9.999999999999998224, 19.99999999999999645 ) ) ;
#15240=CARTESIAN_POINT ( 'NONE',  ( -7.000000000000000000, 8.572527594031473190E-16, 5.000000000000009770 ) ) ;
#15268=DIRECTION ( 'NONE',  ( 0.000000000000000000, 0.000000000000000000, -1.000000000000000000 ) ) ;
#15279=VERTEX_POINT ( 'NONE', #14762 ) ;
#15300=CIRCLE ( 'NONE', #18709, 2.649999999999999467 ) ;
#15301=CARTESIAN_POINT ( 'NONE',  ( -65.00000000000000000, 9.999999999999998224, 17.49999999999999645 ) ) ;
#15337=CARTESIAN_POINT ( 'NONE',  ( -27.50000000000000711, 1.500000000000003109, -33.66025403784446723 ) ) ;
#15340=VECTOR ( 'NONE', #1747, 1000.000000000000000 ) ;
#15342=FACE_BOUND ( 'NONE', #20243, .T. ) ;
#15343=CARTESIAN_POINT ( 'NONE',  ( 54.99999999999992895, 15.00000000000000000, 5.000000000000001776 ) ) ;
#15345=VECTOR ( 'NONE', #2536, 1000.000000000000000 ) ;
#15347=VERTEX_POINT ( 'NONE', #2023 ) ;
#15394=DIRECTION ( 'NONE',  ( -0.000000000000000000, 1.000000000000000000, -0.000000000000000000 ) ) ;
#15412=EDGE_CURVE ( 'NONE', #5919, #2990, #5306, .T. ) ;
#15419=LINE ( 'NONE', #2912, #754 ) ;
#15433=VERTEX_POINT ( 'NONE', #22741 ) ;
#15435=CYLINDRICAL_SURFACE ( 'NONE', #1426, 10.00000000000000178 ) ;
#15448=CARTESIAN_POINT ( 'NONE',  ( -4.898587196589412829E-16, 0.000000000000000000, -4.000000000000000000 ) ) ;
#15450=VERTEX_POINT ( 'NONE', #4310 ) ;
#15457=FACE_OUTER_BOUND ( 'NONE', #15998, .T. ) ;
#15475=DIRECTION ( 'NONE',  ( -1.224646799147353207E-16, 0.000000000000000000, -1.000000000000000000 ) ) ;
#15486=EDGE_LOOP ( 'NONE', ( #18465, #18923, #1933, #7405 ) ) ;
#15527=LINE ( 'NONE', #22564, #22064 ) ;
#15558=CARTESIAN_POINT ( 'NONE',  ( 27.50000000000000000, 1.500000000000003109, -36.31025403784446581 ) ) ;
#15560=CIRCLE ( 'NONE', #19717, 2.500000000000002220 ) ;
#15563=EDGE_LOOP ( 'NONE', ( #16502, #17784 ) ) ;
#15566=EDGE_CURVE ( 'NONE', #20146, #19235, #14143, .T. ) ;
#15576=EDGE_CURVE ( 'NONE', #3743, #3912, #15712, .T. ) ;
#15580=CARTESIAN_POINT ( 'NONE',  ( 35.00000000000000000, 4.500000000000009770, -4.286263797015736496E-15 ) ) ;
#15602=DIRECTION ( 'NONE',  ( -0.000000000000000000, -1.000000000000000000, -0.000000000000000000 ) ) ;
#15604=ORIENTED_EDGE ( 'NONE', *, *, #1471, .F. ) ;
#15611=VERTEX_POINT ( 'NONE', #8515 ) ;
#15621=FACE_OUTER_BOUND ( 'NONE', #3922, .T. ) ;
#15671=EDGE_CURVE ( 'NONE', #22965, #11837, #18332, .T. ) ;
#15672=ADVANCED_FACE ( 'NONE', ( #10081, #16047 ), #15926, .F. ) ;
#15680=MECHANICAL_DESIGN_GEOMETRIC_PRESENTATION_REPRESENTATION('',(#17639),#16480);
#15692=ORIENTED_EDGE ( 'NONE', *, *, #1844, .T. ) ;
#15698=ORIENTED_EDGE ( 'NONE', *, *, #16710, .F. ) ;
#15709=AXIS2_PLACEMENT_3D ( 'NONE', #9998, #17287, #22770 ) ;
#15712=LINE ( 'NONE', #17610, #22531 ) ;
#15730=EDGE_LOOP ( 'NONE', ( #11638, #17213, #897, #6059 ) ) ;
#15796=DIRECTION ( 'NONE',  ( 0.000000000000000000, 0.000000000000000000, 1.000000000000000000 ) ) ;
#15806=EDGE_CURVE ( 'NONE', #17589, #2967, #5714, .T. ) ;
#15813=CARTESIAN_POINT ( 'NONE',  ( 27.50000000000000000, 1.500000000000003109, -36.31025403784446581 ) ) ;
#15817=DIRECTION ( 'NONE',  ( 0.000000000000000000, 0.000000000000000000, -1.000000000000000000 ) ) ;
#15863=ORIENTED_EDGE ( 'NONE', *, *, #1037, .F. ) ;
#15906=LINE ( 'NONE', #1626, #5193 ) ;
#15921=EDGE_CURVE ( 'NONE', #2701, #5919, #20789, .T. ) ;
#15926=PLANE ( 'NONE',  #8401 ) ;
#15927=DIRECTION ( 'NONE',  ( 1.060575238724910366E-16, -0.4999999999999951705, 0.8660254037844414832 ) ) ;
#15942=ORIENTED_EDGE ( 'NONE', *, *, #18920, .F. ) ;
#15947=EDGE_CURVE ( 'NONE', #20420, #16436, #11252, .T. ) ;
#15956=EDGE_CURVE ( 'NONE', #13122, #9843, #13754, .T. ) ;
#15960=LINE ( 'NONE', #19648, #3836 ) ;
#15969=CARTESIAN_POINT ( 'NONE',  ( -27.50000000000000711, 4.500000000000003553, -31.01025403784446510 ) ) ;
#15985=EDGE_CURVE ( 'NONE', #8981, #9536, #15300, .T. ) ;
#15987=AXIS2_PLACEMENT_3D ( 'NONE', #22453, #2223, #74 ) ;
#15988=LINE ( 'NONE', #23274, #4888 ) ;
#15989=VECTOR ( 'NONE', #7902, 1000.000000000000000 ) ;
#15997=CARTESIAN_POINT ( 'NONE',  ( -65.00000000000000000, -10.00000000000000178, 12.49999999999999467 ) ) ;
#15998=EDGE_LOOP ( 'NONE', ( #12522, #6658, #8799, #9654 ) ) ;
#16004=ORIENTED_EDGE ( 'NONE', *, *, #5404, .T. ) ;
#16031=ORIENTED_EDGE ( 'NONE', *, *, #3043, .T. ) ;
#16039=AXIS2_PLACEMENT_3D ( 'NONE', #21574, #4957, #8681 ) ;
#16046=AXIS2_PLACEMENT_3D ( 'NONE', #22844, #13778, #8379 ) ;
#16047=FACE_OUTER_BOUND ( 'NONE', #13842, .T. ) ;
#16052=DIRECTION ( 'NONE',  ( 1.000000000000000000, 4.625929269271486900E-16, -1.224646799147353207E-16 ) ) ;
#16058=SURFACE_STYLE_USAGE ( .BOTH. , #19624 ) ;
#16065=VERTEX_POINT ( 'NONE', #2586 ) ;
#16099=VECTOR ( 'NONE', #15602, 1000.000000000000000 ) ;
#16103=ADVANCED_FACE ( 'NONE', ( #4281, #19236, #8595 ), #4994, .F. ) ;
#16136=ORIENTED_EDGE ( 'NONE', *, *, #17133, .F. ) ;
#16150=EDGE_LOOP ( 'NONE', ( #11630, #19933, #3896, #2539 ) ) ;
#16155=ORIENTED_EDGE ( 'NONE', *, *, #11023, .F. ) ;
#16223=CYLINDRICAL_SURFACE ( 'NONE', #14067, 2.649999999999999467 ) ;
#16239=SURFACE_STYLE_USAGE ( .BOTH. , #21478 ) ;
#16243=CARTESIAN_POINT ( 'NONE',  ( 65.00000000000000000, 15.00000000000000000, 10.00000000000007105 ) ) ;
#16245=VERTEX_POINT ( 'NONE', #13760 ) ;
#16250=DIRECTION ( 'NONE',  ( 0.000000000000000000, 0.000000000000000000, -1.000000000000000000 ) ) ;
#16287=CARTESIAN_POINT ( 'NONE',  ( -20.00000000000000355, -8.499999999999966249, 2.449293598294706907E-15 ) ) ;
#16290=CARTESIAN_POINT ( 'NONE',  ( -60.00000000000000711, -10.00000000000000178, 17.49999999999999645 ) ) ;
#16306=CYLINDRICAL_SURFACE ( 'NONE', #18270, 12.00000000000000000 ) ;
#16330=FACE_OUTER_BOUND ( 'NONE', #15730, .T. ) ;
#16372=DIRECTION ( 'NONE',  ( 0.000000000000000000, 0.000000000000000000, -1.000000000000000000 ) ) ;
#16384=VERTEX_POINT ( 'NONE', #9075 ) ;
#16388=EDGE_CURVE ( 'NONE', #6601, #9734, #3650, .T. ) ;
#16391=DIRECTION ( 'NONE',  ( -1.000000000000000000, 0.000000000000000000, 1.224646799147353207E-16 ) ) ;
#16393=ORIENTED_EDGE ( 'NONE', *, *, #9232, .F. ) ;
#16409=VECTOR ( 'NONE', #6175, 1000.000000000000000 ) ;
#16410=DIRECTION ( 'NONE',  ( 0.000000000000000000, 0.000000000000000000, -1.000000000000000000 ) ) ;
#16423=CIRCLE ( 'NONE', #17573, 2.649999999999999467 ) ;
#16436=VERTEX_POINT ( 'NONE', #1967 ) ;
#16444=CARTESIAN_POINT ( 'NONE',  ( -60.00000000000000711, 15.00000000000000000, 25.00000000000001421 ) ) ;
#16447=ORIENTED_EDGE ( 'NONE', *, *, #10439, .F. ) ;
#16458=CARTESIAN_POINT ( 'NONE',  ( -60.00000000000000711, -9.999999999999998224, 25.00000000000001421 ) ) ;
#16466=ORIENTED_EDGE ( 'NONE', *, *, #7337, .T. ) ;
#16476=DIRECTION ( 'NONE',  ( 1.000000000000000000, 0.000000000000000000, -9.637352644315595243E-17 ) ) ;
#16480=( GEOMETRIC_REPRESENTATION_CONTEXT ( 3 ) GLOBAL_UNCERTAINTY_ASSIGNED_CONTEXT ( ( #3062 ) ) GLOBAL_UNIT_ASSIGNED_CONTEXT ( ( #21533, #1542, #5260 ) ) REPRESENTATION_CONTEXT ( 'NONE', 'WORKASPACE' ) );
#16485=DIRECTION ( 'NONE',  ( -0.000000000000000000, -1.000000000000000000, -0.000000000000000000 ) ) ;
#16501=ORIENTED_EDGE ( 'NONE', *, *, #7350, .F. ) ;
#16502=ORIENTED_EDGE ( 'NONE', *, *, #10889, .T. ) ;
#16511=EDGE_CURVE ( 'NONE', #2967, #15279, #3769, .T. ) ;
#16528=LINE ( 'NONE', #465, #12106 ) ;
#16569=CARTESIAN_POINT ( 'NONE',  ( -9.000000000000000000, 1.102182119232617714E-15, -3.999999999999999112 ) ) ;
#16570=EDGE_CURVE ( 'NONE', #17536, #23404, #17220, .T. ) ;
#16589=ORIENTED_EDGE ( 'NONE', *, *, #17224, .F. ) ;
#16635=ORIENTED_EDGE ( 'NONE', *, *, #3894, .F. ) ;
#16641=AXIS2_PLACEMENT_3D ( 'NONE', #13322, #362, #17137 ) ;
#16669=ORIENTED_EDGE ( 'NONE', *, *, #4603, .T. ) ;
#16677=EDGE_CURVE ( 'NONE', #15450, #6430, #15419, .T. ) ;
#16687=CARTESIAN_POINT ( 'NONE',  ( -60.00000000000000711, 9.999999999999998224, 14.99999999999999645 ) ) ;
#16710=EDGE_CURVE ( 'NONE', #9090, #23518, #17553, .T. ) ;
#16725=ORIENTED_EDGE ( 'NONE', *, *, #15671, .T. ) ;
#16727=AXIS2_PLACEMENT_3D ( 'NONE', #1585, #10734, #20223 ) ;
#16732=ORIENTED_EDGE ( 'NONE', *, *, #547, .F. ) ;
#16748=CIRCLE ( 'NONE', #20928, 12.00000000000000000 ) ;
#16750=VECTOR ( 'NONE', #900, 1000.000000000000000 ) ;
#16764=CARTESIAN_POINT ( 'NONE',  ( -20.00000000000001066, 4.500000000000003553, -50.00000000000000000 ) ) ;
#16797=PLANE ( 'NONE',  #14784 ) ;
#16801=AXIS2_PLACEMENT_3D ( 'NONE', #1058, #2389, #13318 ) ;
#16820=VECTOR ( 'NONE', #7855, 1000.000000000000000 ) ;
#16850=ORIENTED_EDGE ( 'NONE', *, *, #15671, .F. ) ;
#16855=EDGE_CURVE ( 'NONE', #20420, #15433, #22947, .T. ) ;
#16857=EDGE_CURVE ( 'NONE', #19235, #20146, #8439, .T. ) ;
#16884=EDGE_CURVE ( 'NONE', #660, #8473, #5764, .T. ) ;
#16886=ORIENTED_EDGE ( 'NONE', *, *, #1730, .T. ) ;
#16887=DIRECTION ( 'NONE',  ( -1.000000000000000000, 0.000000000000000000, 1.224646799147353207E-16 ) ) ;
#16891=ORIENTED_EDGE ( 'NONE', *, *, #3101, .F. ) ;
#16901=ORIENTED_EDGE ( 'NONE', *, *, #3894, .T. ) ;
#16925=ADVANCED_FACE ( 'NONE', ( #13092 ), #9023, .T. ) ;
#16946=LINE ( 'NONE', #15168, #20179 ) ;
#16951=CARTESIAN_POINT ( 'NONE',  ( 34.99999999999999289, 1.500000000000009992, -50.00000000000000711 ) ) ;
#16955=CYLINDRICAL_SURFACE ( 'NONE', #9717, 2.500000000000002220 ) ;
#16971=CARTESIAN_POINT ( 'NONE',  ( 60.00000000000000000, 9.999999999999998224, 14.99999999999999645 ) ) ;
#17000=DIRECTION ( 'NONE',  ( -0.000000000000000000, -1.000000000000000000, -0.000000000000000000 ) ) ;
#17001=DIRECTION ( 'NONE',  ( -1.224646799147353454E-16, 0.000000000000000000, -1.000000000000000000 ) ) ;
#17035=ORIENTED_EDGE ( 'NONE', *, *, #7610, .F. ) ;
#17044=EDGE_CURVE ( 'NONE', #17175, #9561, #2845, .T. ) ;
#17133=EDGE_CURVE ( 'NONE', #5469, #6601, #6693, .T. ) ;
#17137=DIRECTION ( 'NONE',  ( 1.000000000000000000, 0.000000000000000000, 1.040834085586083271E-15 ) ) ;
#17175=VERTEX_POINT ( 'NONE', #15240 ) ;
#17184=EDGE_CURVE ( 'NONE', #18995, #4822, #9970, .T. ) ;
#17192=LINE ( 'NONE', #16951, #22452 ) ;
#17193=DIRECTION ( 'NONE',  ( -0.000000000000000000, -1.000000000000000000, -0.000000000000000000 ) ) ;
#17213=ORIENTED_EDGE ( 'NONE', *, *, #18986, .F. ) ;
#17218=ORIENTED_EDGE ( 'NONE', *, *, #21059, .T. ) ;
#17220=CIRCLE ( 'NONE', #1889, 7.000000000000000000 ) ;
#17224=EDGE_CURVE ( 'NONE', #2372, #8909, #12001, .T. ) ;
#17232=CIRCLE ( 'NONE', #14564, 2.500000000000002220 ) ;
#17244=VECTOR ( 'NONE', #23126, 1000.000000000000000 ) ;
#17263=CARTESIAN_POINT ( 'NONE',  ( 60.00000000000000711, 9.999999999999998224, 24.99999999999999645 ) ) ;
#17265=ORIENTED_EDGE ( 'NONE', *, *, #18393, .T. ) ;
#17276=ORIENTED_EDGE ( 'NONE', *, *, #3064, .T. ) ;
#17287=DIRECTION ( 'NONE',  ( -1.000000000000000000, 0.000000000000000000, 0.000000000000000000 ) ) ;
#17291=EDGE_CURVE ( 'NONE', #4502, #6195, #1061, .T. ) ;
#17298=ORIENTED_EDGE ( 'NONE', *, *, #4541, .F. ) ;
#17310=ADVANCED_FACE ( 'NONE', ( #13799 ), #19736, .F. ) ;
#17357=DIRECTION ( 'NONE',  ( -1.000000000000000000, 0.000000000000000000, 0.000000000000000000 ) ) ;
#17359=CARTESIAN_POINT ( 'NONE',  ( -60.00000000000000711, 15.00000000000000000, 20.00000000000001421 ) ) ;
#17362=ORIENTED_EDGE ( 'NONE', *, *, #3688, .F. ) ;
#17363=CARTESIAN_POINT ( 'NONE',  ( -65.00000000000000000, 9.999999999999998224, 14.99999999999999645 ) ) ;
#17401=VECTOR ( 'NONE', #16052, 1000.000000000000000 ) ;
#17422=VERTEX_POINT ( 'NONE', #16287 ) ;
#17424=ORIENTED_EDGE ( 'NONE', *, *, #9861, .F. ) ;
#17442=DIRECTION ( 'NONE',  ( -1.224646799147353454E-16, 0.000000000000000000, -1.000000000000000000 ) ) ;
#17473=CARTESIAN_POINT ( 'NONE',  ( 60.00000000000000711, -9.999999999999998224, 24.99999999999999645 ) ) ;
#17475=DIRECTION ( 'NONE',  ( -1.224646799147353207E-16, 0.000000000000000000, -1.000000000000000000 ) ) ;
#17476=DIRECTION ( 'NONE',  ( 0.000000000000000000, 0.000000000000000000, 1.000000000000000000 ) ) ;
#17477=ADVANCED_FACE ( 'NONE', ( #12824 ), #20082, .F. ) ;
#17490=FACE_OUTER_BOUND ( 'NONE', #10400, .T. ) ;
#17494=AXIS2_PLACEMENT_3D ( 'NONE', #1726, #9192, #18258 ) ;
#17495=CARTESIAN_POINT ( 'NONE',  ( -65.00000000000000000, -10.00000000000000178, 14.99999999999999467 ) ) ;
#17536=VERTEX_POINT ( 'NONE', #22236 ) ;
#17545=AXIS2_PLACEMENT_3D ( 'NONE', #5617, #17000, #12949 ) ;
#17553=LINE ( 'NONE', #2802, #21790 ) ;
#17573=AXIS2_PLACEMENT_3D ( 'NONE', #10676, #2971, #5249 ) ;
#17577=ADVANCED_FACE ( 'NONE', ( #15096 ), #22351, .T. ) ;
#17586=LINE ( 'NONE', #10057, #18176 ) ;
#17589=VERTEX_POINT ( 'NONE', #13642 ) ;
#17608=ORIENTED_EDGE ( 'NONE', *, *, #16857, .F. ) ;
#17610=CARTESIAN_POINT ( 'NONE',  ( -65.00000000000000000, -15.00000000000000000, 10.00000000000008882 ) ) ;
#17611=EDGE_CURVE ( 'NONE', #6374, #17685, #7888, .T. ) ;
#17613=EDGE_CURVE ( 'NONE', #9536, #8981, #13227, .T. ) ;
#17634=ORIENTED_EDGE ( 'NONE', *, *, #6263, .T. ) ;
#17639=STYLED_ITEM ( 'NONE', ( #23349 ), #5892 ) ;
#17685=VERTEX_POINT ( 'NONE', #9810 ) ;
#17700=LINE ( 'NONE', #7157, #18193 ) ;
#17705=EDGE_LOOP ( 'NONE', ( #23647, #5723 ) ) ;
#17723=FACE_OUTER_BOUND ( 'NONE', #14934, .T. ) ;
#17745=EDGE_CURVE ( 'NONE', #9843, #1357, #17586, .T. ) ;
#17759=ORIENTED_EDGE ( 'NONE', *, *, #14815, .T. ) ;
#17783=VECTOR ( 'NONE', #21419, 1000.000000000000000 ) ;
#17784=ORIENTED_EDGE ( 'NONE', *, *, #7212, .T. ) ;
#17804=LINE ( 'NONE', #4866, #1670 ) ;
#17805=EDGE_CURVE ( 'NONE', #18995, #22965, #6793, .T. ) ;
#17811=DIRECTION ( 'NONE',  ( -0.000000000000000000, -1.000000000000000000, -0.000000000000000000 ) ) ;
#17814=DIRECTION ( 'NONE',  ( 4.625929269271486900E-16, -1.000000000000000000, -5.665129472695380173E-32 ) ) ;
#17818=DIRECTION ( 'NONE',  ( 1.000000000000000000, -0.000000000000000000, -0.000000000000000000 ) ) ;
#17828=FACE_OUTER_BOUND ( 'NONE', #565, .T. ) ;
#17843=DIRECTION ( 'NONE',  ( 1.000000000000000000, 0.000000000000000000, 0.000000000000000000 ) ) ;
#17928=ORIENTED_EDGE ( 'NONE', *, *, #17613, .T. ) ;
#17940=AXIS2_PLACEMENT_3D ( 'NONE', #17948, #1528, #1879 ) ;
#17945=DIRECTION ( 'NONE',  ( 1.000000000000000000, 0.000000000000000000, 0.000000000000000000 ) ) ;
#17948=CARTESIAN_POINT ( 'NONE',  ( -4.898587196589412829E-16, 0.000000000000000000, -4.000000000000000000 ) ) ;
#17969=EDGE_LOOP ( 'NONE', ( #1043, #18, #19085, #6802 ) ) ;
#17985=DIRECTION ( 'NONE',  ( -0.000000000000000000, -1.000000000000000000, -0.000000000000000000 ) ) ;
#18010=LINE ( 'NONE', #23145, #12163 ) ;
#18015=CARTESIAN_POINT ( 'NONE',  ( -20.00000000000000355, 4.500000000000003553, 2.449293598294706907E-15 ) ) ;
#18049=CARTESIAN_POINT ( 'NONE',  ( 55.00000000000000711, -15.00000000000000000, 10.00000000000000000 ) ) ;
#18050=VERTEX_POINT ( 'NONE', #4016 ) ;
#18084=ORIENTED_EDGE ( 'NONE', *, *, #1004, .F. ) ;
#18099=EDGE_CURVE ( 'NONE', #18050, #4939, #18943, .T. ) ;
#18118=DIRECTION ( 'NONE',  ( -0.000000000000000000, -1.000000000000000000, -0.000000000000000000 ) ) ;
#18176=VECTOR ( 'NONE', #15796, 1000.000000000000000 ) ;
#18193=VECTOR ( 'NONE', #12693, 1000.000000000000000 ) ;
#18209=CARTESIAN_POINT ( 'NONE',  ( -65.00000000000000000, 15.00000000000000000, 20.00000000000001421 ) ) ;
#18220=ORIENTED_EDGE ( 'NONE', *, *, #17613, .F. ) ;
#18222=ORIENTED_EDGE ( 'NONE', *, *, #1037, .T. ) ;
#18252=CARTESIAN_POINT ( 'NONE',  ( 60.00000000000000711, 15.00000000000000000, 10.00000000000007105 ) ) ;
#18258=DIRECTION ( 'NONE',  ( 0.000000000000000000, 0.000000000000000000, -1.000000000000000000 ) ) ;
#18270=AXIS2_PLACEMENT_3D ( 'NONE', #3119, #12613, #19753 ) ;
#18272=VERTEX_POINT ( 'NONE', #22716 ) ;
#18274=CARTESIAN_POINT ( 'NONE',  ( -65.00000000000000000, 9.999999999999998224, 17.49999999999999645 ) ) ;
#18278=ORIENTED_EDGE ( 'NONE', *, *, #18404, .T. ) ;
#18311=DIRECTION ( 'NONE',  ( 1.000000000000000000, 0.000000000000000000, -1.224646799147353207E-16 ) ) ;
#18319=LINE ( 'NONE', #14751, #9167 ) ;
#18322=VECTOR ( 'NONE', #5861, 1000.000000000000000 ) ;
#18326=CYLINDRICAL_SURFACE ( 'NONE', #11081, 2.649999999999999467 ) ;
#18330=EDGE_LOOP ( 'NONE', ( #19453, #22691 ) ) ;
#18332=CIRCLE ( 'NONE', #7650, 5.000000000000000888 ) ;
#18375=DIRECTION ( 'NONE',  ( 1.000000000000000000, 0.000000000000000000, 0.000000000000000000 ) ) ;
#18381=CYLINDRICAL_SURFACE ( 'NONE', #9189, 5.000000000000001776 ) ;
#18393=EDGE_CURVE ( 'NONE', #14895, #3750, #10187, .T. ) ;
#18395=ORIENTED_EDGE ( 'NONE', *, *, #5127, .F. ) ;
#18399=AXIS2_PLACEMENT_3D ( 'NONE', #17495, #22747, #6359 ) ;
#18403=ORIENTED_EDGE ( 'NONE', *, *, #15201, .T. ) ;
#18404=EDGE_CURVE ( 'NONE', #18050, #5914, #12441, .T. ) ;
#18415=DIRECTION ( 'NONE',  ( 1.000000000000000000, 0.000000000000000000, 0.000000000000000000 ) ) ;
#18417=DIRECTION ( 'NONE',  ( 0.000000000000000000, 0.000000000000000000, -1.000000000000000000 ) ) ;
#18418=DIRECTION ( 'NONE',  ( 1.000000000000000000, 0.000000000000000000, -0.000000000000000000 ) ) ;
#18420=EDGE_CURVE ( 'NONE', #4822, #10125, #9038, .T. ) ;
#18424=EDGE_CURVE ( 'NONE', #660, #17422, #8600, .T. ) ;
#18431=EDGE_CURVE ( 'NONE', #13541, #7101, #15906, .T. ) ;
#18465=ORIENTED_EDGE ( 'NONE', *, *, #8231, .F. ) ;
#18466=EDGE_CURVE ( 'NONE', #2990, #22965, #17700, .T. ) ;
#18475=DIRECTION ( 'NONE',  ( 1.000000000000000000, 0.000000000000000000, 0.000000000000000000 ) ) ;
#18490=EDGE_CURVE ( 'NONE', #3871, #6195, #1379, .T. ) ;
#18505=ORIENTED_EDGE ( 'NONE', *, *, #4692, .F. ) ;
#18512=VECTOR ( 'NONE', #15394, 1000.000000000000000 ) ;
#18514=EDGE_LOOP ( 'NONE', ( #3107, #4652, #14608, #13293 ) ) ;
#18526=CARTESIAN_POINT ( 'NONE',  ( 60.00000000000000711, -15.00000000000000000, 10.00000000000007105 ) ) ;
#18537=AXIS2_PLACEMENT_3D ( 'NONE', #20328, #20448, #13184 ) ;
#18574=ORIENTED_EDGE ( 'NONE', *, *, #8231, .T. ) ;
#18627=AXIS2_PLACEMENT_3D ( 'NONE', #12739, #1313, #19989 ) ;
#18628=DIRECTION ( 'NONE',  ( -1.000000000000000000, 0.000000000000000000, 0.000000000000000000 ) ) ;
#18638=ORIENTED_EDGE ( 'NONE', *, *, #1739, .F. ) ;
#18641=STYLED_ITEM ( 'NONE', ( #23168 ), #6561 ) ;
#18650=DIRECTION ( 'NONE',  ( -0.000000000000000000, -1.000000000000000000, -0.000000000000000000 ) ) ;
#18653=DIRECTION ( 'NONE',  ( 0.000000000000000000, 0.000000000000000000, -1.000000000000000000 ) ) ;
#18665=VECTOR ( 'NONE', #5789, 1000.000000000000000 ) ;
#18693=ORIENTED_EDGE ( 'NONE', *, *, #1844, .F. ) ;
#18702=DIRECTION ( 'NONE',  ( 0.000000000000000000, -0.000000000000000000, 1.000000000000000000 ) ) ;
#18709=AXIS2_PLACEMENT_3D ( 'NONE', #13287, #18650, #14851 ) ;
#18717=DIRECTION ( 'NONE',  ( 1.224646799147353207E-16, -0.000000000000000000, 1.000000000000000000 ) ) ;
#18724=EDGE_CURVE ( 'NONE', #15279, #22866, #15560, .T. ) ;
#18755=DIRECTION ( 'NONE',  ( 0.000000000000000000, 0.000000000000000000, 1.000000000000000000 ) ) ;
#18797=ORIENTED_EDGE ( 'NONE', *, *, #21776, .F. ) ;
#18805=DIRECTION ( 'NONE',  ( -1.000000000000000000, 0.000000000000000000, 0.000000000000000000 ) ) ;
#18849=EDGE_LOOP ( 'NONE', ( #19694, #19030, #19276, #18084, #17298, #16901 ) ) ;
#18874=CARTESIAN_POINT ( 'NONE',  ( -20.00000000000000355, 4.500000000000003553, 2.449293598294706907E-15 ) ) ;
#18895=EDGE_LOOP ( 'NONE', ( #6903, #16393, #17276, #13189 ) ) ;
#18920=EDGE_CURVE ( 'NONE', #22617, #5234, #23642, .T. ) ;
#18923=ORIENTED_EDGE ( 'NONE', *, *, #17291, .F. ) ;
#18943=CIRCLE ( 'NONE', #8633, 4.999999999999997335 ) ;
#18956=AXIS2_PLACEMENT_3D ( 'NONE', #7841, #18375, #407 ) ;
#18958=PRODUCT_DEFINITION ( 'UNKNOWN', '', #14909, #13653 ) ;
#18965=DIRECTION ( 'NONE',  ( -1.000000000000000000, 0.000000000000000000, 9.637352644315595243E-17 ) ) ;
#18986=EDGE_CURVE ( 'NONE', #15433, #20420, #4001, .T. ) ;
#18995=VERTEX_POINT ( 'NONE', #14086 ) ;
#19006=CARTESIAN_POINT ( 'NONE',  ( -7.000000000000000000, 8.572527594031473190E-16, 1.734723475976807094E-15 ) ) ;
#19030=ORIENTED_EDGE ( 'NONE', *, *, #20329, .T. ) ;
#19049=EDGE_CURVE ( 'NONE', #15450, #8473, #14445, .T. ) ;
#19067=AXIS2_PLACEMENT_3D ( 'NONE', #3085, #7045, #21505 ) ;
#19084=DIRECTION ( 'NONE',  ( -1.060575238724910366E-16, 0.4999999999999951705, -0.8660254037844414832 ) ) ;
#19085=ORIENTED_EDGE ( 'NONE', *, *, #22071, .F. ) ;
#19112=ORIENTED_EDGE ( 'NONE', *, *, #5127, .T. ) ;
#19133=CYLINDRICAL_SURFACE ( 'NONE', #3271, 2.500000000000002220 ) ;
#19137=FACE_BOUND ( 'NONE', #20325, .T. ) ;
#19151=VECTOR ( 'NONE', #1767, 1000.000000000000000 ) ;
#19158=CARTESIAN_POINT ( 'NONE',  ( 0.000000000000000000, 0.000000000000000000, 5.000000000000008882 ) ) ;
#19235=VERTEX_POINT ( 'NONE', #11804 ) ;
#19236=FACE_BOUND ( 'NONE', #733, .T. ) ;
#19242=ORIENTED_EDGE ( 'NONE', *, *, #23031, .T. ) ;
#19257=DIRECTION ( 'NONE',  ( 1.000000000000000000, -0.000000000000000000, -0.000000000000000000 ) ) ;
#19269=ORIENTED_EDGE ( 'NONE', *, *, #10383, .F. ) ;
#19276=ORIENTED_EDGE ( 'NONE', *, *, #91, .T. ) ;
#19287=CARTESIAN_POINT ( 'NONE',  ( 35.00000000000000000, 1.500000000000009992, -17.32050807568893092 ) ) ;
#19337=ORIENTED_EDGE ( 'NONE', *, *, #112, .F. ) ;
#19359=DIRECTION ( 'NONE',  ( -1.000000000000000000, 0.000000000000000000, 0.000000000000000000 ) ) ;
#19365=VERTEX_POINT ( 'NONE', #10363 ) ;
#19397=ORIENTED_EDGE ( 'NONE', *, *, #16884, .T. ) ;
#19453=ORIENTED_EDGE ( 'NONE', *, *, #4692, .T. ) ;
#19458=VERTEX_POINT ( 'NONE', #11775 ) ;
#19480=ORIENTED_EDGE ( 'NONE', *, *, #9232, .T. ) ;
#19501=AXIS2_PLACEMENT_3D ( 'NONE', #11676, #621, #15268 ) ;
#19518=VERTEX_POINT ( 'NONE', #2753 ) ;
#19548=ORIENTED_EDGE ( 'NONE', *, *, #15956, .T. ) ;
#19563=DIRECTION ( 'NONE',  ( 0.000000000000000000, -0.000000000000000000, 1.000000000000000000 ) ) ;
#19594=FACE_OUTER_BOUND ( 'NONE', #21116, .T. ) ;
#19599=EDGE_CURVE ( 'NONE', #7937, #14895, #8413, .T. ) ;
#19624=SURFACE_SIDE_STYLE ('',( #12362 ) ) ;
#19626=CARTESIAN_POINT ( 'NONE',  ( 54.99999999999992895, -15.00000000000000000, 1.836970198721037478E-15 ) ) ;
#19648=CARTESIAN_POINT ( 'NONE',  ( -20.00000000000000711, 1.500000000000003109, -17.32050807568892736 ) ) ;
#19670=DIRECTION ( 'NONE',  ( 1.000000000000000000, 0.000000000000000000, -0.000000000000000000 ) ) ;
#19681=EDGE_LOOP ( 'NONE', ( #12952, #16725, #9213, #21659, #8274, #8237 ) ) ;
#19687=EDGE_LOOP ( 'NONE', ( #12412, #23439, #16589, #281 ) ) ;
#19694=ORIENTED_EDGE ( 'NONE', *, *, #5896, .T. ) ;
#19705=AXIS2_PLACEMENT_3D ( 'NONE', #12572, #17814, #1514 ) ;
#19717=AXIS2_PLACEMENT_3D ( 'NONE', #20658, #18628, #18755 ) ;
#19726=CARTESIAN_POINT ( 'NONE',  ( 7.000000000000000000, 0.000000000000000000, 5.000000000000007994 ) ) ;
#19736=PLANE ( 'NONE',  #13599 ) ;
#19753=DIRECTION ( 'NONE',  ( 1.000000000000000000, 0.000000000000000000, -1.445602896647339163E-16 ) ) ;
#19759=CARTESIAN_POINT ( 'NONE',  ( 27.50000000000000000, 1.500000000000003109, -31.01025403784446510 ) ) ;
#19781=DIRECTION ( 'NONE',  ( 1.000000000000000000, 3.273063162220391312E-16, 0.000000000000000000 ) ) ;
#19784=LINE ( 'NONE', #14555, #4863 ) ;
#19795=DIRECTION ( 'NONE',  ( 0.000000000000000000, 0.000000000000000000, -1.000000000000000000 ) ) ;
#19835=CARTESIAN_POINT ( 'NONE',  ( 35.00000000000000000, -8.499999999999955591, -4.286263797015736496E-15 ) ) ;
#19840=EDGE_LOOP ( 'NONE', ( #2426, #5176, #16136, #11661 ) ) ;
#19845=ADVANCED_FACE ( 'NONE', ( #1662 ), #5387, .F. ) ;
#19848=CARTESIAN_POINT ( 'NONE',  ( 34.99999999999999289, 4.500000000000009770, -50.00000000000000711 ) ) ;
#19885=DIRECTION ( 'NONE',  ( 0.000000000000000000, 0.000000000000000000, 1.000000000000000000 ) ) ;
#19888=DIRECTION ( 'NONE',  ( -0.000000000000000000, -1.000000000000000000, -0.000000000000000000 ) ) ;
#19894=ORIENTED_EDGE ( 'NONE', *, *, #4103, .T. ) ;
#19904=VERTEX_POINT ( 'NONE', #5854 ) ;
#19912=ADVANCED_FACE ( 'NONE', ( #19137, #4408, #22360, #15342 ), #20912, .T. ) ;
#19921=ORIENTED_EDGE ( 'NONE', *, *, #14924, .T. ) ;
#19933=ORIENTED_EDGE ( 'NONE', *, *, #12290, .T. ) ;
#19983=EDGE_LOOP ( 'NONE', ( #19921, #11235, #18505, #17362 ) ) ;
#19989=DIRECTION ( 'NONE',  ( 0.000000000000000000, 0.000000000000000000, -1.000000000000000000 ) ) ;
#20010=ORIENTED_EDGE ( 'NONE', *, *, #21776, .T. ) ;
#20039=DIRECTION ( 'NONE',  ( 1.000000000000000000, 0.000000000000000000, 0.000000000000000000 ) ) ;
#20054=CARTESIAN_POINT ( 'NONE',  ( 65.00000000000000000, 15.00000000000000000, 24.99999999999999645 ) ) ;
#20074=DIRECTION ( 'NONE',  ( 1.224646799147353207E-16, 0.000000000000000000, 1.000000000000000000 ) ) ;
#20081=CARTESIAN_POINT ( 'NONE',  ( 65.00000000000000000, -10.00000000000000178, 14.99999999999999467 ) ) ;
#20082=PLANE ( 'NONE',  #4393 ) ;
#20088=LINE ( 'NONE', #9590, #5495 ) ;
#20115=ORIENTED_EDGE ( 'NONE', *, *, #18490, .T. ) ;
#20122=CARTESIAN_POINT ( 'NONE',  ( -27.50000000000000711, 1.500000000000003109, -33.66025403784446723 ) ) ;
#20126=AXIS2_PLACEMENT_3D ( 'NONE', #10626, #23516, #12179 ) ;
#20145=CARTESIAN_POINT ( 'NONE',  ( -60.00000000000001421, -9.999999999999998224, 20.00000000000001421 ) ) ;
#20146=VERTEX_POINT ( 'NONE', #21475 ) ;
#20152=LINE ( 'NONE', #5049, #8416 ) ;
#20177=AXIS2_PLACEMENT_3D ( 'NONE', #20639, #4246, #18965 ) ;
#20179=VECTOR ( 'NONE', #6040, 1000.000000000000000 ) ;
#20214=LINE ( 'NONE', #3383, #12938 ) ;
#20221=CIRCLE ( 'NONE', #9938, 2.500000000000002220 ) ;
#20223=DIRECTION ( 'NONE',  ( 1.224646799147353207E-16, 0.000000000000000000, 1.000000000000000000 ) ) ;
#20243=EDGE_LOOP ( 'NONE', ( #726, #11809, #1520, #17035 ) ) ;
#20278=LINE ( 'NONE', #18252, #21704 ) ;
#20293=CARTESIAN_POINT ( 'NONE',  ( -20.00000000000001066, 1.500000000000003109, -50.00000000000000000 ) ) ;
#20297=ORIENTED_EDGE ( 'NONE', *, *, #14815, .F. ) ;
#20325=EDGE_LOOP ( 'NONE', ( #1075, #5208 ) ) ;
#20328=CARTESIAN_POINT ( 'NONE',  ( 54.99999999999992895, 15.00000000000000000, 1.836970198721037478E-15 ) ) ;
#20329=EDGE_CURVE ( 'NONE', #1913, #13267, #13610, .T. ) ;
#20332=DIRECTION ( 'NONE',  ( -0.000000000000000000, -1.000000000000000000, -0.000000000000000000 ) ) ;
#20338=EDGE_CURVE ( 'NONE', #1357, #18995, #6339, .T. ) ;
#20341=EDGE_LOOP ( 'NONE', ( #16155, #11781, #8098, #7819 ) ) ;
#20348=CARTESIAN_POINT ( 'NONE',  ( 55.00000000000000711, -15.00000000000000000, 10.00000000000000000 ) ) ;
#20354=ORIENTED_EDGE ( 'NONE', *, *, #14924, .F. ) ;
#20370=AXIS2_PLACEMENT_3D ( 'NONE', #10707, #17985, #1561 ) ;
#20374=CARTESIAN_POINT ( 'NONE',  ( 19.99999999999999645, 4.500000000000003553, -50.00000000000000000 ) ) ;
#20376=LINE ( 'NONE', #14796, #18665 ) ;
#20382=ORIENTED_EDGE ( 'NONE', *, *, #6137, .F. ) ;
#20419=DIRECTION ( 'NONE',  ( -0.000000000000000000, -1.000000000000000000, -0.000000000000000000 ) ) ;
#20420=VERTEX_POINT ( 'NONE', #15969 ) ;
#20435=CARTESIAN_POINT ( 'NONE',  ( -12.00000000000000000, 1.469576158976823947E-15, -3.999999999999998224 ) ) ;
#20448=DIRECTION ( 'NONE',  ( -1.224646799147353207E-16, 0.000000000000000000, -1.000000000000000000 ) ) ;
#20449=AXIS2_PLACEMENT_3D ( 'NONE', #463, #2725, #16887 ) ;
#20465=EDGE_CURVE ( 'NONE', #1297, #10020, #21815, .T. ) ;
#20499=ADVANCED_FACE ( 'NONE', ( #7820 ), #16797, .F. ) ;
#20504=ADVANCED_FACE ( 'NONE', ( #5777 ), #7709, .T. ) ;
#20534=FACE_OUTER_BOUND ( 'NONE', #18895, .T. ) ;
#20539=CARTESIAN_POINT ( 'NONE',  ( -35.00000000000000711, 16.40063509461079150, -43.12916512459903373 ) ) ;
#20561=DIRECTION ( 'NONE',  ( 1.000000000000000000, -0.000000000000000000, -0.000000000000000000 ) ) ;
#20639=CARTESIAN_POINT ( 'NONE',  ( -4.898587196589412829E-16, 0.000000000000000000, -4.000000000000000000 ) ) ;
#20650=AXIS2_PLACEMENT_3D ( 'NONE', #15337, #22718, #8253 ) ;
#20657=DIRECTION ( 'NONE',  ( 1.000000000000000000, 0.000000000000000000, -4.093947403305266636E-14 ) ) ;
#20658=CARTESIAN_POINT ( 'NONE',  ( -60.00000000000000711, 9.999999999999998224, 14.99999999999999645 ) ) ;
#20682=DIRECTION ( 'NONE',  ( 1.000000000000000000, 0.000000000000000000, -1.445602896647339163E-16 ) ) ;
#20703=ORIENTED_EDGE ( 'NONE', *, *, #15947, .T. ) ;
#20715=LINE ( 'NONE', #2863, #10337 ) ;
#20788=AXIS2_PLACEMENT_3D ( 'NONE', #21489, #5102, #21371 ) ;
#20789=LINE ( 'NONE', #18526, #13774 ) ;
#20792=DIRECTION ( 'NONE',  ( -1.000000000000000000, 0.000000000000000000, 0.000000000000000000 ) ) ;
#20813=CARTESIAN_POINT ( 'NONE',  ( 65.00000000000000000, 9.999999999999998224, 17.49999999999999645 ) ) ;
#20865=ORIENTED_EDGE ( 'NONE', *, *, #23031, .F. ) ;
#20882=ORIENTED_EDGE ( 'NONE', *, *, #4429, .F. ) ;
#20888=CARTESIAN_POINT ( 'NONE',  ( -27.50000000000000711, 1.500000000000003109, -36.31025403784446581 ) ) ;
#20889=CARTESIAN_POINT ( 'NONE',  ( -55.00000000000000000, 15.00000000000000000, 10.00000000000001599 ) ) ;
#20899=AXIS2_PLACEMENT_3D ( 'NONE', #1789, #5278, #10740 ) ;
#20908=CARTESIAN_POINT ( 'NONE',  ( 9.000000000000000000, 0.000000000000000000, -4.000000000000000888 ) ) ;
#20912=PLANE ( 'NONE',  #20449 ) ;
#20914=CARTESIAN_POINT ( 'NONE',  ( 65.00000000000000000, -15.00000000000000000, 10.00000000000007105 ) ) ;
#20919=DIRECTION ( 'NONE',  ( 0.000000000000000000, 0.000000000000000000, -1.000000000000000000 ) ) ;
#20928=AXIS2_PLACEMENT_3D ( 'NONE', #6777, #3293, #12423 ) ;
#20953=DIRECTION ( 'NONE',  ( 1.000000000000000000, -0.000000000000000000, -0.000000000000000000 ) ) ;
#20967=CARTESIAN_POINT ( 'NONE',  ( -60.00000000000000711, 9.999999999999998224, 12.49999999999999289 ) ) ;
#20979=EDGE_LOOP ( 'NONE', ( #16466, #14065, #4906, #3088 ) ) ;
#20988=CARTESIAN_POINT ( 'NONE',  ( -20.00000000000001066, 1.500000000000003109, -50.00000000000000000 ) ) ;
#20991=LINE ( 'NONE', #4610, #23457 ) ;
#21001=DIRECTION ( 'NONE',  ( -0.000000000000000000, -1.000000000000000000, -0.000000000000000000 ) ) ;
#21016=VECTOR ( 'NONE', #11513, 1000.000000000000000 ) ;
#21025=CARTESIAN_POINT ( 'NONE',  ( 65.00000000000000000, 15.00000000000000000, 24.99999999999999645 ) ) ;
#21026=ADVANCED_FACE ( 'NONE', ( #7080, #14395 ), #23108, .T. ) ;
#21033=EDGE_LOOP ( 'NONE', ( #10894, #22280, #5300, #7771, #23326, #3530 ) ) ;
#21036=DIRECTION ( 'NONE',  ( -1.000000000000000000, 0.000000000000000000, 1.224646799147353454E-16 ) ) ;
#21042=ORIENTED_EDGE ( 'NONE', *, *, #6137, .T. ) ;
#21055=DIRECTION ( 'NONE',  ( 1.000000000000000000, 0.000000000000000000, -1.224646799147353207E-16 ) ) ;
#21059=EDGE_CURVE ( 'NONE', #23518, #3912, #18319, .T. ) ;
#21116=EDGE_LOOP ( 'NONE', ( #13212, #14581, #6202, #19242 ) ) ;
#21122=EDGE_CURVE ( 'NONE', #6430, #15019, #2012, .T. ) ;
#21203=ORIENTED_EDGE ( 'NONE', *, *, #18424, .F. ) ;
#21211=VECTOR ( 'NONE', #5967, 1000.000000000000000 ) ;
#21240=CIRCLE ( 'NONE', #3656, 10.00000000000000178 ) ;
#21245=UNCERTAINTY_MEASURE_WITH_UNIT (LENGTH_MEASURE( 1.000000000000000082E-05 ), #21286, 'distance_accuracy_value', 'NONE');
#21249=EDGE_LOOP ( 'NONE', ( #11025, #14327, #11341, #16501 ) ) ;
#21254=DIRECTION ( 'NONE',  ( -0.000000000000000000, -1.000000000000000000, -0.000000000000000000 ) ) ;
#21284=CARTESIAN_POINT ( 'NONE',  ( -55.00000000000000000, -15.00000000000000000, 10.00000000000001599 ) ) ;
#21286=( LENGTH_UNIT ( ) NAMED_UNIT ( * ) SI_UNIT ( .MILLI., .METRE. ) );
#21293=DIRECTION ( 'NONE',  ( -1.224646799147353207E-16, 0.000000000000000000, -1.000000000000000000 ) ) ;
#21371=DIRECTION ( 'NONE',  ( 0.000000000000000000, 0.000000000000000000, 1.000000000000000000 ) ) ;
#21383=DIRECTION ( 'NONE',  ( -1.060575238724910366E-16, 0.4999999999999951150, -0.8660254037844414832 ) ) ;
#21387=PLANE ( 'NONE',  #19067 ) ;
#21391=ORIENTED_EDGE ( 'NONE', *, *, #21122, .F. ) ;
#21397=AXIS2_PLACEMENT_3D ( 'NONE', #3044, #17442, #10035 ) ;
#21403=DIRECTION ( 'NONE',  ( 0.000000000000000000, -1.000000000000000000, 0.000000000000000000 ) ) ;
#21407=CIRCLE ( 'NONE', #22571, 2.500000000000002220 ) ;
#21415=( NAMED_UNIT ( * ) PLANE_ANGLE_UNIT ( ) SI_UNIT ( $, .RADIAN. ) );
#21419=DIRECTION ( 'NONE',  ( 1.000000000000000000, -0.000000000000000000, -0.000000000000000000 ) ) ;
#21436=CARTESIAN_POINT ( 'NONE',  ( 34.99999999999999289, 4.500000000000009770, -50.00000000000000711 ) ) ;
#21462=DIRECTION ( 'NONE',  ( -0.000000000000000000, -1.000000000000000000, -0.000000000000000000 ) ) ;
#21471=VERTEX_POINT ( 'NONE', #6688 ) ;
#21475=CARTESIAN_POINT ( 'NONE',  ( 12.00000000000000000, 0.000000000000000000, -4.000000000000001776 ) ) ;
#21476=ORIENTED_EDGE ( 'NONE', *, *, #18431, .F. ) ;
#21478=SURFACE_SIDE_STYLE ('',( #21598 ) ) ;
#21488=AXIS2_PLACEMENT_3D ( 'NONE', #4877, #10658, #8376 ) ;
#21489=CARTESIAN_POINT ( 'NONE',  ( -55.00000000000000000, 15.00000000000000000, 10.00000000000001599 ) ) ;
#21499=CARTESIAN_POINT ( 'NONE',  ( 54.99999999999992895, -8.499999999999966249, 1.836970198721037478E-15 ) ) ;
#21505=DIRECTION ( 'NONE',  ( -0.000000000000000000, 0.000000000000000000, -1.000000000000000000 ) ) ;
#21533=( LENGTH_UNIT ( ) NAMED_UNIT ( * ) SI_UNIT ( .MILLI., .METRE. ) );
#21570=VECTOR ( 'NONE', #7131, 1000.000000000000000 ) ;
#21574=CARTESIAN_POINT ( 'NONE',  ( 55.00000000000000711, -15.00000000000000000, 10.00000000000000000 ) ) ;
#21598=SURFACE_STYLE_FILL_AREA ( #12549 ) ;
#21601=CARTESIAN_POINT ( 'NONE',  ( -55.00000000000000000, 15.00000000000000000, 10.00000000000001599 ) ) ;
#21617=VECTOR ( 'NONE', #6572, 1000.000000000000000 ) ;
#21632=EDGE_LOOP ( 'NONE', ( #20297, #5269 ) ) ;
#21638=PLANE ( 'NONE',  #12568 ) ;
#21639=DIRECTION ( 'NONE',  ( 1.000000000000000000, 0.000000000000000000, -0.000000000000000000 ) ) ;
#21652=( NAMED_UNIT ( * ) SI_UNIT ( $, .STERADIAN. ) SOLID_ANGLE_UNIT ( ) );
#21656=CARTESIAN_POINT ( 'NONE',  ( -65.00000000000000000, 9.999999999999998224, 12.49999999999999289 ) ) ;
#21659=ORIENTED_EDGE ( 'NONE', *, *, #3176, .F. ) ;
#21667=CARTESIAN_POINT ( 'NONE',  ( 27.50000000000000000, 1.500000000000003109, -31.01025403784446510 ) ) ;
#21688=MECHANICAL_DESIGN_GEOMETRIC_PRESENTATION_REPRESENTATION('',(#18641),#4504);
#21689=AXIS2_PLACEMENT_3D ( 'NONE', #5301, #3260, #19781 ) ;
#21702=CARTESIAN_POINT ( 'NONE',  ( 27.50000000000000000, 1.500000000000003109, -33.66025403784446723 ) ) ;
#21704=VECTOR ( 'NONE', #13132, 1000.000000000000000 ) ;
#21739=DIRECTION ( 'NONE',  ( -1.000000000000000000, -4.625929269271486900E-16, 0.000000000000000000 ) ) ;
#21755=( GEOMETRIC_REPRESENTATION_CONTEXT ( 3 ) GLOBAL_UNCERTAINTY_ASSIGNED_CONTEXT ( ( #21245 ) ) GLOBAL_UNIT_ASSIGNED_CONTEXT ( ( #21286, #21415, #21652 ) ) REPRESENTATION_CONTEXT ( 'NONE', 'WORKASPACE' ) );
#21769=VECTOR ( 'NONE', #16485, 1000.000000000000000 ) ;
#21776=EDGE_CURVE ( 'NONE', #19904, #9536, #2351, .T. ) ;
#21790=VECTOR ( 'NONE', #23040, 1000.000000000000000 ) ;
#21791=FACE_OUTER_BOUND ( 'NONE', #10131, .T. ) ;
#21794=FACE_OUTER_BOUND ( 'NONE', #106, .T. ) ;
#21795=AXIS2_PLACEMENT_3D ( 'NONE', #20054, #3659, #5582 ) ;
#21811=ORIENTED_EDGE ( 'NONE', *, *, #5699, .F. ) ;
#21815=LINE ( 'NONE', #3381, #3261 ) ;
#21875=CARTESIAN_POINT ( 'NONE',  ( 54.99999999999992895, -15.00000000000000000, 1.836970198721037478E-15 ) ) ;
#21892=DIRECTION ( 'NONE',  ( 0.000000000000000000, 0.000000000000000000, 1.000000000000000000 ) ) ;
#21905=DIRECTION ( 'NONE',  ( 1.224646799147353207E-16, -0.000000000000000000, 1.000000000000000000 ) ) ;
#21915=VERTEX_POINT ( 'NONE', #10283 ) ;
#21925=DIRECTION ( 'NONE',  ( 1.000000000000000000, 0.000000000000000000, 0.000000000000000000 ) ) ;
#21951=ADVANCED_FACE ( 'NONE', ( #3418 ), #18381, .F. ) ;
#21956=ADVANCED_FACE ( 'NONE', ( #1841 ), #10760, .F. ) ;
#21980=ORIENTED_EDGE ( 'NONE', *, *, #4066, .F. ) ;
#21988=CARTESIAN_POINT ( 'NONE',  ( 65.00000000000000000, -10.00000000000000178, 14.99999999999999467 ) ) ;
#22009=ORIENTED_EDGE ( 'NONE', *, *, #4832, .F. ) ;
#22013=CARTESIAN_POINT ( 'NONE',  ( 27.50000000000000000, 1.500000000000003109, -33.66025403784446723 ) ) ;
#22024=DIRECTION ( 'NONE',  ( -1.000000000000000000, 0.000000000000000000, 1.224646799147352961E-16 ) ) ;
#22045=ADVANCED_FACE ( 'NONE', ( #23417, #7021, #23654 ), #1725, .T. ) ;
#22052=CARTESIAN_POINT ( 'NONE',  ( 65.00000000000000000, 15.00000000000000000, 19.99999999999999645 ) ) ;
#22064=VECTOR ( 'NONE', #6172, 1000.000000000000000 ) ;
#22068=VECTOR ( 'NONE', #5826, 1000.000000000000000 ) ;
#22071=EDGE_CURVE ( 'NONE', #1297, #5303, #20152, .T. ) ;
#22104=AXIS2_PLACEMENT_3D ( 'NONE', #9208, #11484, #430 ) ;
#22109=CARTESIAN_POINT ( 'NONE',  ( -65.00000000000000000, 9.999999999999998224, 14.99999999999999645 ) ) ;
#22136=DIRECTION ( 'NONE',  ( 1.000000000000000000, -0.000000000000000000, -0.000000000000000000 ) ) ;
#22220=ORIENTED_EDGE ( 'NONE', *, *, #16857, .T. ) ;
#22232=DIRECTION ( 'NONE',  ( -0.000000000000000000, -1.000000000000000000, -0.000000000000000000 ) ) ;
#22236=CARTESIAN_POINT ( 'NONE',  ( 7.000000000000000000, 0.000000000000000000, 1.734723475976807094E-15 ) ) ;
#22247=DIRECTION ( 'NONE',  ( -1.224646799147353207E-16, 0.000000000000000000, -1.000000000000000000 ) ) ;
#22273=EDGE_LOOP ( 'NONE', ( #18395, #6461, #23202, #811 ) ) ;
#22280=ORIENTED_EDGE ( 'NONE', *, *, #15412, .T. ) ;
#22318=CARTESIAN_POINT ( 'NONE',  ( 0.000000000000000000, 0.000000000000000000, 1.734723475976807094E-15 ) ) ;
#22335=DIRECTION ( 'NONE',  ( -0.000000000000000000, -1.000000000000000000, -0.000000000000000000 ) ) ;
#22351=CYLINDRICAL_SURFACE ( 'NONE', #3263, 12.00000000000000000 ) ;
#22360=FACE_BOUND ( 'NONE', #10220, .T. ) ;
#22392=CIRCLE ( 'NONE', #2111, 5.000000000000000888 ) ;
#22401=ORIENTED_EDGE ( 'NONE', *, *, #20465, .F. ) ;
#22434=CARTESIAN_POINT ( 'NONE',  ( -55.00000000000000000, -15.00000000000000000, 10.00000000000001599 ) ) ;
#22450=ORIENTED_EDGE ( 'NONE', *, *, #19599, .T. ) ;
#22452=VECTOR ( 'NONE', #13848, 1000.000000000000000 ) ;
#22453=CARTESIAN_POINT ( 'NONE',  ( -27.50000000000000711, 1.500000000000003109, -33.66025403784446723 ) ) ;
#22458=VECTOR ( 'NONE', #17818, 1000.000000000000000 ) ;
#22475=EDGE_LOOP ( 'NONE', ( #4874, #5007, #19548, #304 ) ) ;
#22477=VERTEX_POINT ( 'NONE', #6767 ) ;
#22480=ORIENTED_EDGE ( 'NONE', *, *, #19049, .F. ) ;
#22484=CARTESIAN_POINT ( 'NONE',  ( -6.123233995736766085E-15, 0.000000000000000000, -50.00000000000000000 ) ) ;
#22488=ORIENTED_EDGE ( 'NONE', *, *, #5404, .F. ) ;
#22493=VECTOR ( 'NONE', #12215, 1000.000000000000000 ) ;
#22497=ADVANCED_FACE ( 'NONE', ( #4618 ), #2560, .T. ) ;
#22511=DIRECTION ( 'NONE',  ( -1.224646799147353207E-16, 0.000000000000000000, -1.000000000000000000 ) ) ;
#22515=ORIENTED_EDGE ( 'NONE', *, *, #1201, .F. ) ;
#22531=VECTOR ( 'NONE', #15817, 1000.000000000000000 ) ;
#22564=CARTESIAN_POINT ( 'NONE',  ( 54.99999999999992895, 15.00000000000000000, 5.000000000000001776 ) ) ;
#22571=AXIS2_PLACEMENT_3D ( 'NONE', #2721, #20561, #4166 ) ;
#22597=ADVANCED_FACE ( 'NONE', ( #9176, #23513 ), #5548, .F. ) ;
#22614=LINE ( 'NONE', #13780, #15989 ) ;
#22617=VERTEX_POINT ( 'NONE', #7373 ) ;
#22641=EDGE_LOOP ( 'NONE', ( #1237, #14883, #18638, #11573, #10999, #17218 ) ) ;
#22691=ORIENTED_EDGE ( 'NONE', *, *, #7350, .T. ) ;
#22698=CARTESIAN_POINT ( 'NONE',  ( -65.00000000000000000, 15.00000000000000000, 10.00000000000008882 ) ) ;
#22715=DIRECTION ( 'NONE',  ( 1.224646799147353207E-16, -0.000000000000000000, 1.000000000000000000 ) ) ;
#22716=CARTESIAN_POINT ( 'NONE',  ( -65.00000000000000000, -10.00000000000000178, 17.49999999999999645 ) ) ;
#22718=DIRECTION ( 'NONE',  ( -0.000000000000000000, -1.000000000000000000, -0.000000000000000000 ) ) ;
#22734=VECTOR ( 'NONE', #3048, 1000.000000000000000 ) ;
#22740=ORIENTED_EDGE ( 'NONE', *, *, #4635, .F. ) ;
#22741=CARTESIAN_POINT ( 'NONE',  ( -27.50000000000000711, 4.500000000000003553, -36.31025403784446581 ) ) ;
#22747=DIRECTION ( 'NONE',  ( 1.000000000000000000, -0.000000000000000000, -0.000000000000000000 ) ) ;
#22770=DIRECTION ( 'NONE',  ( 0.000000000000000000, 0.000000000000000000, 1.000000000000000000 ) ) ;
#22844=CARTESIAN_POINT ( 'NONE',  ( -60.00000000000000711, 9.999999999999998224, 20.00000000000001421 ) ) ;
#22858=DIRECTION ( 'NONE',  ( 0.000000000000000000, -0.000000000000000000, -1.000000000000000000 ) ) ;
#22866=VERTEX_POINT ( 'NONE', #20967 ) ;
#22918=PLANE ( 'NONE',  #10688 ) ;
#22939=ORIENTED_EDGE ( 'NONE', *, *, #9236, .F. ) ;
#22941=FACE_BOUND ( 'NONE', #2406, .T. ) ;
#22947=CIRCLE ( 'NONE', #6514, 2.649999999999999467 ) ;
#22965=VERTEX_POINT ( 'NONE', #10004 ) ;
#22967=PLANE ( 'NONE',  #12977 ) ;
#22968=FACE_OUTER_BOUND ( 'NONE', #16150, .T. ) ;
#22976=EDGE_CURVE ( 'NONE', #4822, #2990, #1210, .T. ) ;
#23031=EDGE_CURVE ( 'NONE', #10020, #19518, #8086, .T. ) ;
#23040=DIRECTION ( 'NONE',  ( 0.000000000000000000, 0.000000000000000000, -1.000000000000000000 ) ) ;
#23054=PLANE ( 'NONE',  #10258 ) ;
#23061=VECTOR ( 'NONE', #18717, 1000.000000000000000 ) ;
#23088=ORIENTED_EDGE ( 'NONE', *, *, #20329, .F. ) ;
#23108=PLANE ( 'NONE',  #14402 ) ;
#23124=CARTESIAN_POINT ( 'NONE',  ( 20.00000000000000355, -8.499999999999962697, 6.123233995736764507E-15 ) ) ;
#23126=DIRECTION ( 'NONE',  ( 1.000000000000000000, 0.000000000000000000, -1.224646799147353207E-16 ) ) ;
#23127=EDGE_CURVE ( 'NONE', #21471, #22617, #4991, .T. ) ;
#23129=ORIENTED_EDGE ( 'NONE', *, *, #2736, .F. ) ;
#23138=VECTOR ( 'NONE', #14391, 1000.000000000000000 ) ;
#23145=CARTESIAN_POINT ( 'NONE',  ( -27.50000000000000711, 1.500000000000003109, -36.31025403784446581 ) ) ;
#23148=CARTESIAN_POINT ( 'NONE',  ( 65.00000000000000000, 15.00000000000000000, 10.00000000000007105 ) ) ;
#23153=AXIS2_PLACEMENT_3D ( 'NONE', #18049, #14596, #3657 ) ;
#23160=LINE ( 'NONE', #4971, #3323 ) ;
#23168=PRESENTATION_STYLE_ASSIGNMENT (( #16239 ) ) ;
#23174=EDGE_LOOP ( 'NONE', ( #15863, #19112, #4973, #9101 ) ) ;
#23178=DIRECTION ( 'NONE',  ( 0.000000000000000000, 0.000000000000000000, 1.000000000000000000 ) ) ;
#23184=ORIENTED_EDGE ( 'NONE', *, *, #17044, .T. ) ;
#23187=LINE ( 'NONE', #8604, #10068 ) ;
#23202=ORIENTED_EDGE ( 'NONE', *, *, #8530, .T. ) ;
#23206=CIRCLE ( 'NONE', #17545, 2.649999999999999467 ) ;
#23215=FILL_AREA_STYLE_COLOUR ( '', #13822 ) ;
#23233=EDGE_CURVE ( 'NONE', #9734, #5914, #23373, .T. ) ;
#23234=DIRECTION ( 'NONE',  ( -0.000000000000000000, -1.000000000000000000, -0.000000000000000000 ) ) ;
#23241=DIRECTION ( 'NONE',  ( 0.000000000000000000, 0.000000000000000000, -1.000000000000000000 ) ) ;
#23274=CARTESIAN_POINT ( 'NONE',  ( -65.00000000000000000, -10.00000000000000178, 17.49999999999999645 ) ) ;
#23282=LINE ( 'NONE', #6769, #11395 ) ;
#23322=CARTESIAN_POINT ( 'NONE',  ( -65.00000000000000000, -15.00000000000000000, 10.00000000000008882 ) ) ;
#23326=ORIENTED_EDGE ( 'NONE', *, *, #15106, .F. ) ;
#23327=VECTOR ( 'NONE', #14475, 1000.000000000000000 ) ;
#23349=PRESENTATION_STYLE_ASSIGNMENT (( #16058 ) ) ;
#23367=LINE ( 'NONE', #6971, #770 ) ;
#23373=LINE ( 'NONE', #14542, #17244 ) ;
#23387=EDGE_LOOP ( 'NONE', ( #9218, #22220 ) ) ;
#23390=DIRECTION ( 'NONE',  ( -0.000000000000000000, -1.000000000000000000, -0.000000000000000000 ) ) ;
#23404=VERTEX_POINT ( 'NONE', #13097 ) ;
#23417=FACE_BOUND ( 'NONE', #13844, .T. ) ;
#23439=ORIENTED_EDGE ( 'NONE', *, *, #4635, .T. ) ;
#23457=VECTOR ( 'NONE', #7979, 1000.000000000000000 ) ;
#23465=EDGE_CURVE ( 'NONE', #13122, #14895, #600, .T. ) ;
#23473=DIRECTION ( 'NONE',  ( 1.000000000000000000, 0.000000000000000000, 0.000000000000000000 ) ) ;
#23477=FACE_OUTER_BOUND ( 'NONE', #19983, .T. ) ;
#23485=DIRECTION ( 'NONE',  ( 1.224646799147353207E-16, -0.000000000000000000, 1.000000000000000000 ) ) ;
#23496=AXIS2_PLACEMENT_3D ( 'NONE', #20081, #18418, #1997 ) ;
#23513=FACE_BOUND ( 'NONE', #7561, .T. ) ;
#23516=DIRECTION ( 'NONE',  ( 0.000000000000000000, 0.000000000000000000, 1.000000000000000000 ) ) ;
#23518=VERTEX_POINT ( 'NONE', #6241 ) ;
#23532=DIRECTION ( 'NONE',  ( -0.000000000000000000, -1.000000000000000000, -0.000000000000000000 ) ) ;
#23558=FACE_BOUND ( 'NONE', #3557, .T. ) ;
#23567=EDGE_CURVE ( 'NONE', #589, #17422, #20715, .T. ) ;
#23586=ORIENTED_EDGE ( 'NONE', *, *, #7212, .F. ) ;
#23621=ORIENTED_EDGE ( 'NONE', *, *, #7164, .T. ) ;
#23635=CIRCLE ( 'NONE', #5275, 2.500000000000002220 ) ;
#23642=LINE ( 'NONE', #15997, #21570 ) ;
#23647=ORIENTED_EDGE ( 'NONE', *, *, #18986, .T. ) ;
#23654=FACE_OUTER_BOUND ( 'NONE', #19681, .T. ) ;
#23691=EDGE_LOOP ( 'NONE', ( #17424, #16886, #14615, #979 ) ) ;
#23696=CIRCLE ( 'NONE', #13772, 2.500000000000000444 ) ;
ENDSEC;
END-ISO-10303-21;
